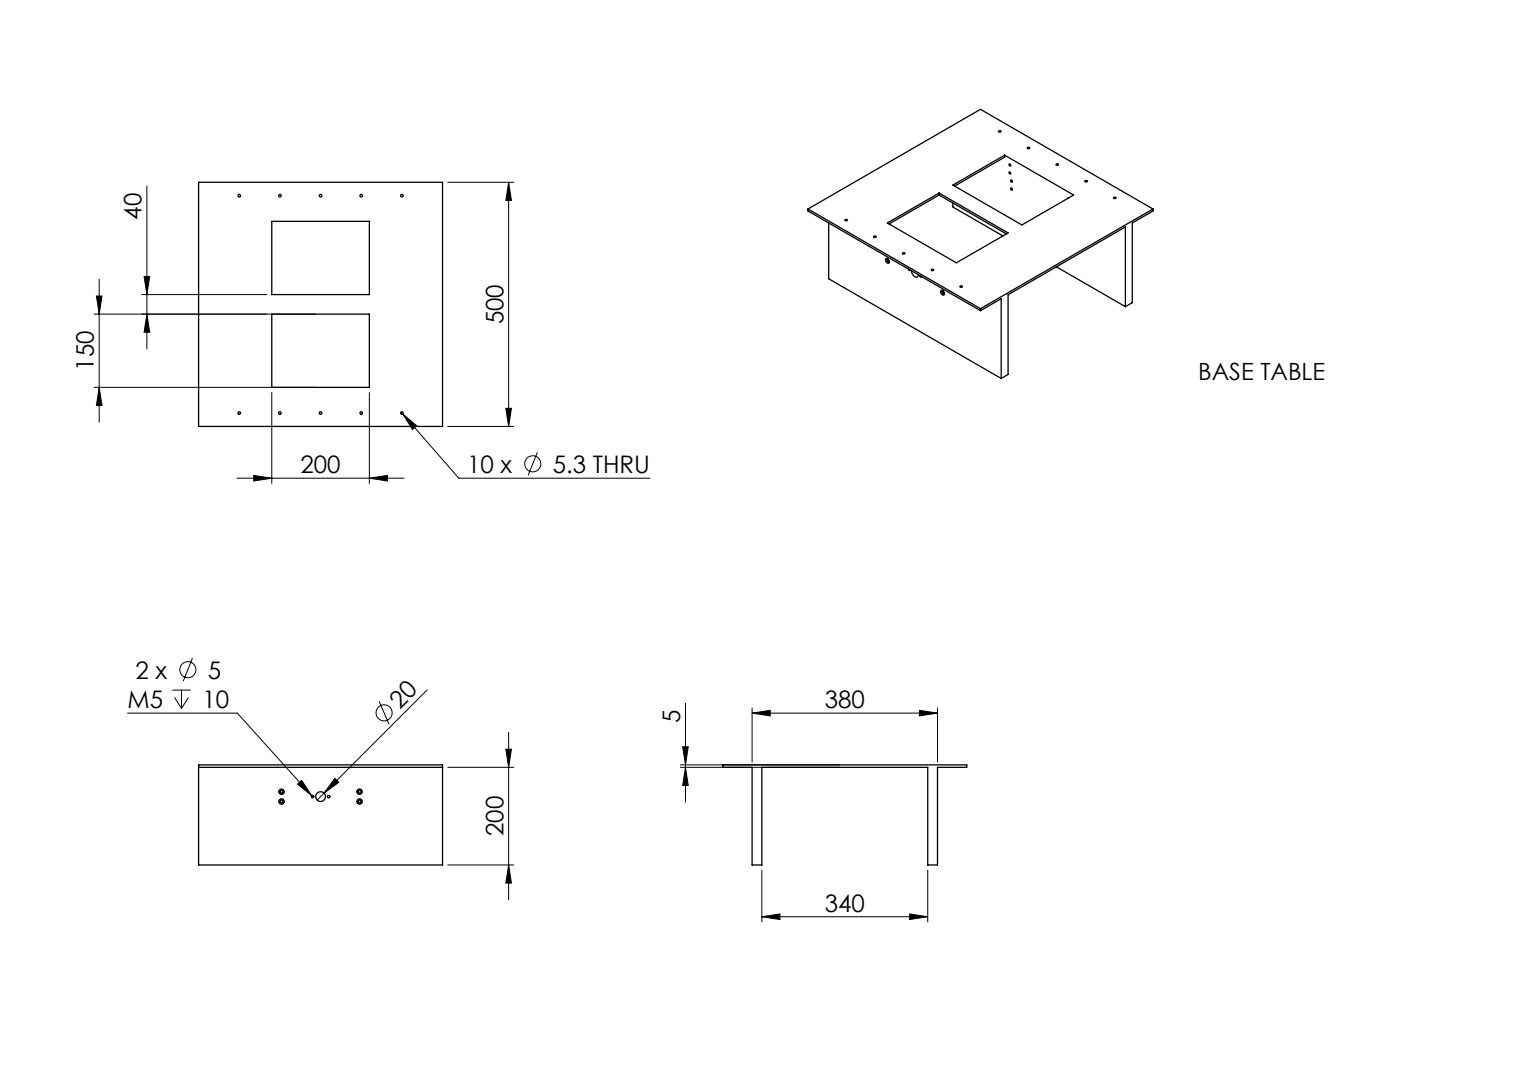
ISO-10303-21;
HEADER;
FILE_DESCRIPTION (('STEP AP214'),
    '1' );
FILE_NAME ('base table.step',
    '2026-10-24T13:33:06',
    ( '' ),
    ( '' ),
    'SwSTEP 2.0',
    'SolidWorks 2026',
    '' );
FILE_SCHEMA (( 'AUTOMOTIVE_DESIGN' ));
ENDSEC;

DATA;
#1=CARTESIAN_POINT ( 'NONE',  ( 53.33333333333330017, -25.00000000000000000, 222.5000000000000853 ) ) ;
#3=ORIENTED_EDGE ( 'NONE', *, *, #4024, .T. ) ;
#4=CARTESIAN_POINT ( 'NONE',  ( 302.6499999999999204, -75.00000000000008527, 169.9999999999999716 ) ) ;
#5=CARTESIAN_POINT ( 'NONE',  ( 136.6666666666666288, -20.00000000000000000, -219.8500000000001080 ) ) ;
#12=LINE ( 'NONE', #10262, #8342 ) ;
#13=LINE ( 'NONE', #14246, #12970 ) ;
#19=DIRECTION ( 'NONE',  ( 1.000000000000000000, 0.000000000000000000, 0.000000000000000000 ) ) ;
#22=CARTESIAN_POINT ( 'NONE',  ( 137.4999999999999432, -36.99999999999997868, -180.0000000000000000 ) ) ;
#29=CARTESIAN_POINT ( 'NONE',  ( 302.6499999999999204, -75.00000000000008527, 186.2999999999999829 ) ) ;
#36=ORIENTED_EDGE ( 'NONE', *, *, #2375, .F. ) ;
#40=ORIENTED_EDGE ( 'NONE', *, *, #13656, .T. ) ;
#44=DIRECTION ( 'NONE',  ( -0.000000000000000000, -0.000000000000000000, 1.000000000000000000 ) ) ;
#45=CARTESIAN_POINT ( 'NONE',  ( 386.6666666666666288, -20.00000000000000000, 225.1500000000000625 ) ) ;
#47=CARTESIAN_POINT ( 'NONE',  ( -30.00000000000002842, -25.00000000000000000, 250.0000000000000000 ) ) ;
#51=ORIENTED_EDGE ( 'NONE', *, *, #14217, .F. ) ;
#52=FACE_OUTER_BOUND ( 'NONE', #5422, .T. ) ;
#65=CARTESIAN_POINT ( 'NONE',  ( -30.00000000000002842, -20.00000000000000000, 250.0000000000000000 ) ) ;
#70=DIRECTION ( 'NONE',  ( 0.000000000000000000, 1.000000000000000000, 0.000000000000000000 ) ) ;
#76=LINE ( 'NONE', #7062, #6983 ) ;
#85=EDGE_CURVE ( 'NONE', #6756, #11518, #12060, .T. ) ;
#86=ADVANCED_FACE ( 'NONE', ( #14292 ), #14148, .F. ) ;
#90=ORIENTED_EDGE ( 'NONE', *, *, #8678, .T. ) ;
#96=ORIENTED_EDGE ( 'NONE', *, *, #5946, .F. ) ;
#107=LINE ( 'NONE', #12182, #1892 ) ;
#108=LINE ( 'NONE', #6679, #5937 ) ;
#111=CARTESIAN_POINT ( 'NONE',  ( 132.4999999999999432, -36.99999999999997868, -169.9999999999999716 ) ) ;
#113=CIRCLE ( 'NONE', #1517, 5.500000000000005329 ) ;
#119=CARTESIAN_POINT ( 'NONE',  ( 134.5000000000000000, -95.00000000000008527, 190.0000000000000000 ) ) ;
#122=LINE ( 'NONE', #2191, #4564 ) ;
#124=CARTESIAN_POINT ( 'NONE',  ( 142.6500000000000057, -95.00000000000008527, 190.0000000000000000 ) ) ;
#134=VECTOR ( 'NONE', #9384, 1000.000000000000000 ) ;
#138=VECTOR ( 'NONE', #5329, 1000.000000000000000 ) ;
#144=VECTOR ( 'NONE', #12485, 1000.000000000000000 ) ;
#164=EDGE_CURVE ( 'NONE', #13531, #14219, #11463, .T. ) ;
#173=PRODUCT ( 'base table', 'base table', '', ( #338 ) ) ;
#177=CIRCLE ( 'NONE', #2061, 2.500000000000002220 ) ;
#178=ORIENTED_EDGE ( 'NONE', *, *, #7566, .F. ) ;
#180=CARTESIAN_POINT ( 'NONE',  ( 299.9999999999999432, -95.00000000000008527, 190.0000000000000000 ) ) ;
#181=CARTESIAN_POINT ( 'NONE',  ( 302.6499999999999204, -95.00000000000008527, -186.2999999999999829 ) ) ;
#183=VECTOR ( 'NONE', #12816, 1000.000000000000000 ) ;
#186=DIRECTION ( 'NONE',  ( 1.000000000000000000, 0.000000000000000000, 0.000000000000000000 ) ) ;
#190=EDGE_LOOP ( 'NONE', ( #1618, #1963 ) ) ;
#192=CARTESIAN_POINT ( 'NONE',  ( 303.3333333333333144, -20.00000000000000000, -219.8500000000001080 ) ) ;
#193=ORIENTED_EDGE ( 'NONE', *, *, #7276, .F. ) ;
#195=CIRCLE ( 'NONE', #13619, 2.500000000000002220 ) ;
#196=EDGE_LOOP ( 'NONE', ( #178, #7479, #11699, #10408 ) ) ;
#197=DIRECTION ( 'NONE',  ( -0.000000000000000000, -0.000000000000000000, -1.000000000000000000 ) ) ;
#201=CARTESIAN_POINT ( 'NONE',  ( 294.4999999999999432, -75.00000000000008527, -190.0000000000000000 ) ) ;
#207=DIRECTION ( 'NONE',  ( 0.000000000000000000, -0.000000000000000000, 1.000000000000000000 ) ) ;
#211=ORIENTED_EDGE ( 'NONE', *, *, #1146, .F. ) ;
#223=LINE ( 'NONE', #12223, #5365 ) ;
#228=AXIS2_PLACEMENT_3D ( 'NONE', #3013, #14095, #2869 ) ;
#229=DIRECTION ( 'NONE',  ( -0.000000000000000000, -0.000000000000000000, -1.000000000000000000 ) ) ;
#234=EDGE_CURVE ( 'NONE', #10453, #9107, #4526, .T. ) ;
#244=ADVANCED_FACE ( 'NONE', ( #3220 ), #6544, .F. ) ;
#252=CARTESIAN_POINT ( 'NONE',  ( 307.5000000000000000, -56.99999999999997158, -180.0000000000000000 ) ) ;
#255=CARTESIAN_POINT ( 'NONE',  ( 119.9999999999999147, -20.00000000000000000, 19.99999999999998934 ) ) ;
#262=DIRECTION ( 'NONE',  ( -1.000000000000000000, 0.000000000000000000, 0.000000000000000000 ) ) ;
#265=ORIENTED_EDGE ( 'NONE', *, *, #11090, .F. ) ;
#266=EDGE_CURVE ( 'NONE', #11339, #3317, #13546, .T. ) ;
#267=CARTESIAN_POINT ( 'NONE',  ( 319.9999999999999432, -225.0010000000000048, 19.99999999999998934 ) ) ;
#268=ORIENTED_EDGE ( 'NONE', *, *, #5003, .F. ) ;
#279=ORIENTED_EDGE ( 'NONE', *, *, #5164, .T. ) ;
#288=DIRECTION ( 'NONE',  ( 0.000000000000000000, 0.000000000000000000, 1.000000000000000000 ) ) ;
#290=DIRECTION ( 'NONE',  ( -0.000000000000000000, 1.000000000000000000, -0.000000000000000000 ) ) ;
#293=EDGE_CURVE ( 'NONE', #12041, #2215, #4727, .T. ) ;
#295=CARTESIAN_POINT ( 'NONE',  ( 302.6499999999999204, -75.00000000000008527, 186.2999999999999829 ) ) ;
#299=DIRECTION ( 'NONE',  ( -0.000000000000000000, -0.000000000000000000, 1.000000000000000000 ) ) ;
#319=ORIENTED_EDGE ( 'NONE', *, *, #6736, .T. ) ;
#320=EDGE_LOOP ( 'NONE', ( #13311, #10317 ) ) ;
#322=AXIS2_PLACEMENT_3D ( 'NONE', #13350, #6899, #4588 ) ;
#325=CARTESIAN_POINT ( 'NONE',  ( 142.6500000000000057, -75.00000000000008527, 186.2999999999999829 ) ) ;
#326=EDGE_CURVE ( 'NONE', #2746, #3344, #2466, .T. ) ;
#328=VERTEX_POINT ( 'NONE', #3699 ) ;
#330=ORIENTED_EDGE ( 'NONE', *, *, #1288, .T. ) ;
#331=DIRECTION ( 'NONE',  ( 0.000000000000000000, 0.000000000000000000, 1.000000000000000000 ) ) ;
#336=CIRCLE ( 'NONE', #815, 5.500000000000005329 ) ;
#338=PRODUCT_CONTEXT ( 'NONE', #6572, 'mechanical' ) ;
#342=FACE_BOUND ( 'NONE', #10311, .T. ) ;
#347=ORIENTED_EDGE ( 'NONE', *, *, #12633, .T. ) ;
#357=DIRECTION ( 'NONE',  ( 1.000000000000000000, 0.000000000000000000, 0.000000000000000000 ) ) ;
#358=CARTESIAN_POINT ( 'NONE',  ( -30.00000000000002842, -225.0000000000000000, -169.9999999999999716 ) ) ;
#363=CIRCLE ( 'NONE', #6654, 2.649999999999985700 ) ;
#364=ORIENTED_EDGE ( 'NONE', *, *, #6973, .T. ) ;
#365=VECTOR ( 'NONE', #9606, 1000.000000000000000 ) ;
#366=VECTOR ( 'NONE', #12284, 1000.000000000000000 ) ;
#375=CARTESIAN_POINT ( 'NONE',  ( 132.4999999999999432, -56.99999999999997158, -180.0000000000000000 ) ) ;
#380=VECTOR ( 'NONE', #10926, 1000.000000000000000 ) ;
#381=DIRECTION ( 'NONE',  ( 0.000000000000000000, 0.000000000000000000, -1.000000000000000000 ) ) ;
#383=ADVANCED_FACE ( 'NONE', ( #52 ), #4580, .F. ) ;
#385=DIRECTION ( 'NONE',  ( -1.000000000000000000, 0.000000000000000000, 0.000000000000000000 ) ) ;
#390=CARTESIAN_POINT ( 'NONE',  ( 302.6499999999999204, -95.00000000000008527, -169.9999999999999716 ) ) ;
#391=CARTESIAN_POINT ( 'NONE',  ( 134.5000000000000000, -95.00000000000008527, -190.0000000000000000 ) ) ;
#398=EDGE_LOOP ( 'NONE', ( #3253, #13729, #3961, #12497 ) ) ;
#405=DIRECTION ( 'NONE',  ( 0.000000000000000000, 0.000000000000000000, -1.000000000000000000 ) ) ;
#409=FACE_BOUND ( 'NONE', #9655, .T. ) ;
#412=CARTESIAN_POINT ( 'NONE',  ( 140.0000000000000000, -75.00000000000008527, 186.2999999999999829 ) ) ;
#430=DIRECTION ( 'NONE',  ( -0.000000000000000000, -0.000000000000000000, 1.000000000000000000 ) ) ;
#434=EDGE_CURVE ( 'NONE', #8157, #4114, #1575, .T. ) ;
#439=( NAMED_UNIT ( * ) PLANE_ANGLE_UNIT ( ) SI_UNIT ( $, .RADIAN. ) );
#445=ORIENTED_EDGE ( 'NONE', *, *, #2431, .F. ) ;
#446=ADVANCED_FACE ( 'NONE', ( #13984, #8328 ), #12831, .F. ) ;
#453=AXIS2_PLACEMENT_3D ( 'NONE', #6130, #4839, #11360 ) ;
#464=CARTESIAN_POINT ( 'NONE',  ( 53.33333333333330017, -20.00000000000000000, -222.5000000000000853 ) ) ;
#474=ORIENTED_EDGE ( 'NONE', *, *, #10554, .T. ) ;
#481=CARTESIAN_POINT ( 'NONE',  ( 219.9999999999999716, -20.00000000000000000, -222.5000000000000853 ) ) ;
#504=EDGE_CURVE ( 'NONE', #1416, #12143, #787, .T. ) ;
#505=DIRECTION ( 'NONE',  ( 0.000000000000000000, 1.000000000000000000, 0.000000000000000000 ) ) ;
#511=DIRECTION ( 'NONE',  ( -1.000000000000000000, 0.000000000000000000, 0.000000000000000000 ) ) ;
#523=DIRECTION ( 'NONE',  ( 1.000000000000000000, 0.000000000000000000, 0.000000000000000000 ) ) ;
#525=DIRECTION ( 'NONE',  ( 1.000000000000000000, 0.000000000000000000, 0.000000000000000000 ) ) ;
#530=EDGE_CURVE ( 'NONE', #11552, #6716, #8218, .T. ) ;
#533=CYLINDRICAL_SURFACE ( 'NONE', #8092, 5.500000000000005329 ) ;
#541=CARTESIAN_POINT ( 'NONE',  ( 299.9999999999999432, -75.00000000000008527, -186.2999999999999829 ) ) ;
#552=AXIS2_PLACEMENT_3D ( 'NONE', #1164, #6764, #11129 ) ;
#563=SHAPE_DEFINITION_REPRESENTATION ( #6804, #2740 ) ;
#567=CIRCLE ( 'NONE', #11715, 5.500000000000005329 ) ;
#569=ORIENTED_EDGE ( 'NONE', *, *, #1110, .T. ) ;
#577=DIRECTION ( 'NONE',  ( -1.000000000000000000, 0.000000000000000000, 0.000000000000000000 ) ) ;
#580=CARTESIAN_POINT ( 'NONE',  ( 142.6500000000000057, -75.00000000000008527, 190.0000000000000000 ) ) ;
#581=CARTESIAN_POINT ( 'NONE',  ( -30.00000000000002842, -25.00000000000000000, -190.0000000000000000 ) ) ;
#582=VECTOR ( 'NONE', #10152, 1000.000000000000000 ) ;
#595=CIRCLE ( 'NONE', #10589, 2.649999999999985700 ) ;
#601=CIRCLE ( 'NONE', #4808, 5.500000000000005329 ) ;
#604=DIRECTION ( 'NONE',  ( 0.000000000000000000, 0.000000000000000000, -1.000000000000000000 ) ) ;
#614=EDGE_CURVE ( 'NONE', #1243, #10967, #14200, .T. ) ;
#624=FACE_OUTER_BOUND ( 'NONE', #10767, .T. ) ;
#626=CIRCLE ( 'NONE', #2277, 2.649999999999985700 ) ;
#627=EDGE_LOOP ( 'NONE', ( #3, #5676 ) ) ;
#630=FACE_OUTER_BOUND ( 'NONE', #8470, .T. ) ;
#634=VERTEX_POINT ( 'NONE', #11963 ) ;
#639=ADVANCED_FACE ( 'NONE', ( #12036 ), #6380, .T. ) ;
#641=CARTESIAN_POINT ( 'NONE',  ( 134.5000000000000000, -95.00000000000008527, 186.2999999999999829 ) ) ;
#647=EDGE_LOOP ( 'NONE', ( #6758, #1729, #6097, #8404 ) ) ;
#654=ORIENTED_EDGE ( 'NONE', *, *, #11946, .F. ) ;
#657=FACE_OUTER_BOUND ( 'NONE', #3143, .T. ) ;
#660=VECTOR ( 'NONE', #9403, 1000.000000000000000 ) ;
#665=EDGE_CURVE ( 'NONE', #10366, #9474, #11020, .T. ) ;
#668=CARTESIAN_POINT ( 'NONE',  ( 297.3499999999999659, -75.00000000000008527, 190.0000000000000000 ) ) ;
#670=CARTESIAN_POINT ( 'NONE',  ( 53.33333333333330017, -20.00000000000000000, 219.8500000000001080 ) ) ;
#677=ORIENTED_EDGE ( 'NONE', *, *, #85, .T. ) ;
#680=AXIS2_PLACEMENT_3D ( 'NONE', #9201, #13616, #5933 ) ;
#684=ADVANCED_FACE ( 'NONE', ( #12904 ), #1050, .F. ) ;
#687=CARTESIAN_POINT ( 'NONE',  ( 386.6666666666666288, -20.00000000000000000, -225.1500000000000625 ) ) ;
#691=DIRECTION ( 'NONE',  ( 1.000000000000000000, 0.000000000000000000, 0.000000000000000000 ) ) ;
#693=EDGE_CURVE ( 'NONE', #6913, #7861, #567, .T. ) ;
#699=ORIENTED_EDGE ( 'NONE', *, *, #13846, .F. ) ;
#701=VERTEX_POINT ( 'NONE', #8913 ) ;
#704=EDGE_CURVE ( 'NONE', #9413, #1808, #6868, .T. ) ;
#712=DIRECTION ( 'NONE',  ( -1.000000000000000000, 0.000000000000000000, 0.000000000000000000 ) ) ;
#715=ORIENTED_EDGE ( 'NONE', *, *, #13042, .T. ) ;
#716=EDGE_CURVE ( 'NONE', #12041, #2872, #7875, .T. ) ;
#721=CARTESIAN_POINT ( 'NONE',  ( 303.3333333333333144, -20.00000000000000000, 222.5000000000000853 ) ) ;
#724=ORIENTED_EDGE ( 'NONE', *, *, #9957, .F. ) ;
#732=DIRECTION ( 'NONE',  ( -1.000000000000000000, 0.000000000000000000, -0.000000000000000000 ) ) ;
#736=ORIENTED_EDGE ( 'NONE', *, *, #1947, .F. ) ;
#738=ORIENTED_EDGE ( 'NONE', *, *, #5484, .T. ) ;
#746=FACE_OUTER_BOUND ( 'NONE', #11832, .T. ) ;
#750=DIRECTION ( 'NONE',  ( -0.000000000000000000, 1.000000000000000000, -0.000000000000000000 ) ) ;
#751=ORIENTED_EDGE ( 'NONE', *, *, #4831, .F. ) ;
#761=LINE ( 'NONE', #8324, #11554 ) ;
#768=LINE ( 'NONE', #3270, #2096 ) ;
#770=VERTEX_POINT ( 'NONE', #6803 ) ;
#782=CARTESIAN_POINT ( 'NONE',  ( 307.5000000000000000, -56.99999999999997158, -169.9999999999999716 ) ) ;
#787=CIRCLE ( 'NONE', #4296, 2.649999999999985700 ) ;
#789=ORIENTED_EDGE ( 'NONE', *, *, #12859, .T. ) ;
#798=CARTESIAN_POINT ( 'NONE',  ( 319.9999999999999432, -20.00000000000000000, -169.9999999999999716 ) ) ;
#800=EDGE_CURVE ( 'NONE', #11046, #2569, #4631, .T. ) ;
#801=AXIS2_PLACEMENT_3D ( 'NONE', #6751, #6960, #5730 ) ;
#804=FACE_OUTER_BOUND ( 'NONE', #5648, .T. ) ;
#805=ORIENTED_EDGE ( 'NONE', *, *, #11640, .F. ) ;
#812=FACE_BOUND ( 'NONE', #4854, .T. ) ;
#815=AXIS2_PLACEMENT_3D ( 'NONE', #8559, #2026, #7322 ) ;
#816=DIRECTION ( 'NONE',  ( 0.000000000000000000, 1.000000000000000000, 0.000000000000000000 ) ) ;
#823=CARTESIAN_POINT ( 'NONE',  ( 134.9999999999999432, -56.99999999999997158, -181.5021515430661054 ) ) ;
#826=CARTESIAN_POINT ( 'NONE',  ( 302.6499999999999204, -95.00000000000008527, 186.2999999999999829 ) ) ;
#828=AXIS2_PLACEMENT_3D ( 'NONE', #1488, #13687, #385 ) ;
#832=CIRCLE ( 'NONE', #6862, 2.649999999999985700 ) ;
#833=FACE_OUTER_BOUND ( 'NONE', #7177, .T. ) ;
#835=CARTESIAN_POINT ( 'NONE',  ( 145.5000000000000284, -95.00000000000008527, -186.2999999999999829 ) ) ;
#840=VERTEX_POINT ( 'NONE', #10067 ) ;
#842=CARTESIAN_POINT ( 'NONE',  ( 470.0000000000000000, -25.00000000000000000, 190.0000000000000000 ) ) ;
#845=ORIENTED_EDGE ( 'NONE', *, *, #3733, .F. ) ;
#857=ORIENTED_EDGE ( 'NONE', *, *, #8071, .F. ) ;
#861=CARTESIAN_POINT ( 'NONE',  ( 142.6500000000000057, -75.00000000000008527, 169.9999999999999716 ) ) ;
#868=LINE ( 'NONE', #3158, #1741 ) ;
#871=EDGE_CURVE ( 'NONE', #1382, #840, #5112, .T. ) ;
#872=EDGE_CURVE ( 'NONE', #10300, #5386, #4179, .T. ) ;
#878=EDGE_CURVE ( 'NONE', #10453, #5579, #6146, .T. ) ;
#881=CYLINDRICAL_SURFACE ( 'NONE', #3412, 2.649999999999985700 ) ;
#887=CYLINDRICAL_SURFACE ( 'NONE', #1179, 5.500000000000005329 ) ;
#893=AXIS2_PLACEMENT_3D ( 'NONE', #8075, #11492, #13514 ) ;
#897=DIRECTION ( 'NONE',  ( -0.8571673013836870192, 1.049727191973306873E-16, 0.5150380737757234151 ) ) ;
#899=CYLINDRICAL_SURFACE ( 'NONE', #1302, 2.649999999999985700 ) ;
#908=FACE_OUTER_BOUND ( 'NONE', #5250, .T. ) ;
#912=ORIENTED_EDGE ( 'NONE', *, *, #1614, .T. ) ;
#918=PLANE ( 'NONE',  #2210 ) ;
#932=CARTESIAN_POINT ( 'NONE',  ( 206.0000000000000284, -85.00000000000007105, 190.0000000000000000 ) ) ;
#936=CIRCLE ( 'NONE', #6523, 2.649999999999985700 ) ;
#940=EDGE_CURVE ( 'NONE', #5316, #11325, #10663, .T. ) ;
#942=CARTESIAN_POINT ( 'NONE',  ( 303.3333333333333144, -20.00000000000000000, -222.5000000000000853 ) ) ;
#945=VECTOR ( 'NONE', #1140, 1000.000000000000000 ) ;
#947=EDGE_CURVE ( 'NONE', #11046, #13697, #12507, .T. ) ;
#948=DIRECTION ( 'NONE',  ( 0.000000000000000000, 0.000000000000000000, 1.000000000000000000 ) ) ;
#950=ADVANCED_FACE ( 'NONE', ( #2663 ), #533, .F. ) ;
#951=ORIENTED_EDGE ( 'NONE', *, *, #6482, .F. ) ;
#967=CARTESIAN_POINT ( 'NONE',  ( 386.6666666666666288, -25.00000000000000000, -225.1500000000000625 ) ) ;
#969=VECTOR ( 'NONE', #7214, 1000.000000000000000 ) ;
#982=CARTESIAN_POINT ( 'NONE',  ( 119.9999999999999147, -225.0010000000000048, 169.9999999999999716 ) ) ;
#989=DIRECTION ( 'NONE',  ( -0.000000000000000000, -0.000000000000000000, 1.000000000000000000 ) ) ;
#991=CARTESIAN_POINT ( 'NONE',  ( 305.0000000000000000, -56.99999999999997158, -180.0000000000000000 ) ) ;
#993=DIRECTION ( 'NONE',  ( -0.000000000000000000, 0.000000000000000000, 1.000000000000000000 ) ) ;
#995=CARTESIAN_POINT ( 'NONE',  ( 132.4999999999999432, -56.99999999999997158, -169.9999999999999716 ) ) ;
#1000=CARTESIAN_POINT ( 'NONE',  ( 307.5000000000000000, -36.99999999999997868, -180.0000000000000000 ) ) ;
#1001=EDGE_LOOP ( 'NONE', ( #951, #1693, #8534, #1264, #9691, #5453, #13384, #1955 ) ) ;
#1006=VERTEX_POINT ( 'NONE', #967 ) ;
#1009=DIRECTION ( 'NONE',  ( -0.000000000000000000, -0.000000000000000000, 1.000000000000000000 ) ) ;
#1012=CARTESIAN_POINT ( 'NONE',  ( 136.6666666666666288, -20.00000000000000000, 222.5000000000000853 ) ) ;
#1013=CARTESIAN_POINT ( 'NONE',  ( -30.00000000000002842, -25.00000000000000000, 169.9999999999999716 ) ) ;
#1020=VERTEX_POINT ( 'NONE', #9776 ) ;
#1023=EDGE_LOOP ( 'NONE', ( #4597, #2682 ) ) ;
#1025=PLANE ( 'NONE',  #13721 ) ;
#1027=AXIS2_PLACEMENT_3D ( 'NONE', #5838, #6852, #3593 ) ;
#1028=ORIENTED_EDGE ( 'NONE', *, *, #4301, .T. ) ;
#1035=AXIS2_PLACEMENT_3D ( 'NONE', #3051, #5502, #14059 ) ;
#1048=ORIENTED_EDGE ( 'NONE', *, *, #6214, .T. ) ;
#1050=CYLINDRICAL_SURFACE ( 'NONE', #1035, 2.649999999999985700 ) ;
#1053=DIRECTION ( 'NONE',  ( -0.000000000000000000, 0.000000000000000000, -1.000000000000000000 ) ) ;
#1056=EDGE_CURVE ( 'NONE', #13697, #10145, #8756, .T. ) ;
#1065=DIRECTION ( 'NONE',  ( -0.000000000000000000, -1.000000000000000000, -0.000000000000000000 ) ) ;
#1066=AXIS2_PLACEMENT_3D ( 'NONE', #12203, #2342, #2270 ) ;
#1068=CYLINDRICAL_SURFACE ( 'NONE', #8248, 5.500000000000005329 ) ;
#1072=ORIENTED_EDGE ( 'NONE', *, *, #85, .F. ) ;
#1075=AXIS2_PLACEMENT_3D ( 'NONE', #7410, #2850, #7263 ) ;
#1080=EDGE_CURVE ( 'NONE', #14253, #2215, #14042, .T. ) ;
#1086=CIRCLE ( 'NONE', #12451, 2.500000000000002220 ) ;
#1091=( LENGTH_UNIT ( ) NAMED_UNIT ( * ) SI_UNIT ( .MILLI., .METRE. ) );
#1095=DIRECTION ( 'NONE',  ( 0.000000000000000000, 0.000000000000000000, -1.000000000000000000 ) ) ;
#1096=ORIENTED_EDGE ( 'NONE', *, *, #3247, .F. ) ;
#1101=CYLINDRICAL_SURFACE ( 'NONE', #5026, 2.649999999999985700 ) ;
#1109=DIRECTION ( 'NONE',  ( -0.000000000000000000, 1.000000000000000000, -0.000000000000000000 ) ) ;
#1110=EDGE_CURVE ( 'NONE', #8867, #8759, #4189, .T. ) ;
#1117=ORIENTED_EDGE ( 'NONE', *, *, #9700, .F. ) ;
#1118=LINE ( 'NONE', #2643, #11978 ) ;
#1120=DIRECTION ( 'NONE',  ( -0.000000000000000000, -0.000000000000000000, -1.000000000000000000 ) ) ;
#1125=VERTEX_POINT ( 'NONE', #823 ) ;
#1131=ORIENTED_EDGE ( 'NONE', *, *, #12517, .F. ) ;
#1132=ORIENTED_EDGE ( 'NONE', *, *, #2253, .T. ) ;
#1134=DIRECTION ( 'NONE',  ( -1.000000000000000000, 0.000000000000000000, 0.000000000000000000 ) ) ;
#1138=AXIS2_PLACEMENT_3D ( 'NONE', #13702, #10598, #12689 ) ;
#1140=DIRECTION ( 'NONE',  ( -0.000000000000000000, 1.000000000000000000, -0.000000000000000000 ) ) ;
#1141=DIRECTION ( 'NONE',  ( -0.000000000000000000, -0.000000000000000000, 1.000000000000000000 ) ) ;
#1146=EDGE_CURVE ( 'NONE', #10315, #11952, #6039, .T. ) ;
#1152=VECTOR ( 'NONE', #8133, 1000.000000000000000 ) ;
#1154=EDGE_CURVE ( 'NONE', #3317, #2814, #8816, .T. ) ;
#1159=VECTOR ( 'NONE', #2534, 1000.000000000000000 ) ;
#1164=CARTESIAN_POINT ( 'NONE',  ( 140.0000000000000000, -75.00000000000008527, 186.2999999999999829 ) ) ;
#1168=ADVANCED_FACE ( 'NONE', ( #13249 ), #9988, .F. ) ;
#1169=EDGE_CURVE ( 'NONE', #1125, #9107, #13723, .T. ) ;
#1172=EDGE_LOOP ( 'NONE', ( #1315, #8576 ) ) ;
#1173=ADVANCED_FACE ( 'NONE', ( #9235, #6910 ), #3583, .F. ) ;
#1176=ORIENTED_EDGE ( 'NONE', *, *, #293, .F. ) ;
#1179=AXIS2_PLACEMENT_3D ( 'NONE', #10929, #10718, #7581 ) ;
#1181=DIRECTION ( 'NONE',  ( -0.000000000000000000, 0.000000000000000000, 1.000000000000000000 ) ) ;
#1183=CARTESIAN_POINT ( 'NONE',  ( 294.4999999999999432, -75.00000000000008527, -190.0000000000000000 ) ) ;
#1186=DIRECTION ( 'NONE',  ( -0.000000000000000000, 1.000000000000000000, -0.000000000000000000 ) ) ;
#1187=CARTESIAN_POINT ( 'NONE',  ( 299.9999999999999432, -75.00000000000008527, -186.2999999999999829 ) ) ;
#1189=LINE ( 'NONE', #5768, #6517 ) ;
#1192=CARTESIAN_POINT ( 'NONE',  ( 470.0000000000000000, -25.00000000000000000, 250.0000000000000000 ) ) ;
#1193=ADVANCED_FACE ( 'NONE', ( #9918 ), #9336, .F. ) ;
#1194=ORIENTED_EDGE ( 'NONE', *, *, #2773, .T. ) ;
#1195=CARTESIAN_POINT ( 'NONE',  ( 305.4999999999999432, -95.00000000000008527, 186.2999999999999829 ) ) ;
#1199=FACE_OUTER_BOUND ( 'NONE', #9157, .T. ) ;
#1202=AXIS2_PLACEMENT_3D ( 'NONE', #11836, #12995, #2993 ) ;
#1203=ORIENTED_EDGE ( 'NONE', *, *, #5421, .T. ) ;
#1205=( NAMED_UNIT ( * ) SI_UNIT ( $, .STERADIAN. ) SOLID_ANGLE_UNIT ( ) );
#1210=ORIENTED_EDGE ( 'NONE', *, *, #9443, .F. ) ;
#1215=DIRECTION ( 'NONE',  ( -0.000000000000000000, -0.000000000000000000, 1.000000000000000000 ) ) ;
#1216=DIRECTION ( 'NONE',  ( -0.000000000000000000, -0.000000000000000000, 1.000000000000000000 ) ) ;
#1220=DIRECTION ( 'NONE',  ( 0.000000000000000000, 0.000000000000000000, -1.000000000000000000 ) ) ;
#1224=ORIENTED_EDGE ( 'NONE', *, *, #3247, .T. ) ;
#1226=ORIENTED_EDGE ( 'NONE', *, *, #3673, .F. ) ;
#1230=ORIENTED_EDGE ( 'NONE', *, *, #4069, .T. ) ;
#1231=PLANE ( 'NONE',  #3603 ) ;
#1243=VERTEX_POINT ( 'NONE', #9159 ) ;
#1252=EDGE_CURVE ( 'NONE', #3125, #6716, #11626, .T. ) ;
#1260=CARTESIAN_POINT ( 'NONE',  ( 136.6666666666666288, -25.00000000000000000, 222.5000000000000853 ) ) ;
#1264=ORIENTED_EDGE ( 'NONE', *, *, #4414, .T. ) ;
#1266=DIRECTION ( 'NONE',  ( -1.000000000000000000, 0.000000000000000000, 0.000000000000000000 ) ) ;
#1281=LINE ( 'NONE', #5721, #945 ) ;
#1286=AXIS2_PLACEMENT_3D ( 'NONE', #9219, #6100, #8120 ) ;
#1287=ORIENTED_EDGE ( 'NONE', *, *, #13354, .T. ) ;
#1288=EDGE_CURVE ( 'NONE', #1020, #2372, #9042, .T. ) ;
#1291=CARTESIAN_POINT ( 'NONE',  ( 470.0000000000000000, -20.00000000000000000, 250.0000000000000000 ) ) ;
#1293=ORIENTED_EDGE ( 'NONE', *, *, #9936, .T. ) ;
#1295=VECTOR ( 'NONE', #505, 1000.000000000000000 ) ;
#1297=DIRECTION ( 'NONE',  ( 0.000000000000000000, 0.000000000000000000, -1.000000000000000000 ) ) ;
#1302=AXIS2_PLACEMENT_3D ( 'NONE', #4049, #7521, #1864 ) ;
#1306=CARTESIAN_POINT ( 'NONE',  ( -30.00000000000002842, -25.00000000000000000, 250.0000000000000000 ) ) ;
#1313=ORIENTED_EDGE ( 'NONE', *, *, #13261, .T. ) ;
#1315=ORIENTED_EDGE ( 'NONE', *, *, #12071, .F. ) ;
#1323=EDGE_CURVE ( 'NONE', #3167, #3720, #9507, .T. ) ;
#1333=DIRECTION ( 'NONE',  ( 0.000000000000000000, 1.000000000000000000, 0.000000000000000000 ) ) ;
#1343=EDGE_CURVE ( 'NONE', #6665, #8094, #10619, .T. ) ;
#1348=EDGE_LOOP ( 'NONE', ( #3565, #1722 ) ) ;
#1349=CARTESIAN_POINT ( 'NONE',  ( 203.5000000000000000, -85.00000000000007105, 180.0000000000000000 ) ) ;
#1352=ORIENTED_EDGE ( 'NONE', *, *, #13379, .F. ) ;
#1369=ORIENTED_EDGE ( 'NONE', *, *, #12633, .F. ) ;
#1370=FACE_OUTER_BOUND ( 'NONE', #7900, .T. ) ;
#1371=ORIENTED_EDGE ( 'NONE', *, *, #13161, .F. ) ;
#1372=CIRCLE ( 'NONE', #11351, 2.649999999999985700 ) ;
#1373=DIRECTION ( 'NONE',  ( -0.000000000000000000, -0.000000000000000000, 1.000000000000000000 ) ) ;
#1374=CARTESIAN_POINT ( 'NONE',  ( 299.9999999999999432, -95.00000000000008527, 186.2999999999999829 ) ) ;
#1380=CARTESIAN_POINT ( 'NONE',  ( 238.9999999999999432, -85.00000000000007105, 190.0000000000000000 ) ) ;
#1381=VERTEX_POINT ( 'NONE', #6113 ) ;
#1382=VERTEX_POINT ( 'NONE', #5186 ) ;
#1389=ORIENTED_EDGE ( 'NONE', *, *, #13899, .T. ) ;
#1390=DIRECTION ( 'NONE',  ( 1.000000000000000000, 0.000000000000000000, 0.000000000000000000 ) ) ;
#1397=FACE_OUTER_BOUND ( 'NONE', #9178, .T. ) ;
#1404=DIRECTION ( 'NONE',  ( -1.000000000000000000, 0.000000000000000000, 0.000000000000000000 ) ) ;
#1407=EDGE_LOOP ( 'NONE', ( #8578, #7757, #9815, #9066 ) ) ;
#1408=AXIS2_PLACEMENT_3D ( 'NONE', #6574, #5477, #9911 ) ;
#1415=EDGE_CURVE ( 'NONE', #6044, #3377, #11120, .T. ) ;
#1416=VERTEX_POINT ( 'NONE', #3365 ) ;
#1418=AXIS2_PLACEMENT_3D ( 'NONE', #10970, #3355, #2105 ) ;
#1422=EDGE_LOOP ( 'NONE', ( #10256, #6078 ) ) ;
#1442=CARTESIAN_POINT ( 'NONE',  ( 470.0000000000000000, -25.00000000000000000, 250.0000000000000000 ) ) ;
#1447=DIRECTION ( 'NONE',  ( -1.000000000000000000, 0.000000000000000000, 0.000000000000000000 ) ) ;
#1448=VERTEX_POINT ( 'NONE', #12062 ) ;
#1449=CYLINDRICAL_SURFACE ( 'NONE', #13340, 2.649999999999985700 ) ;
#1451=DIRECTION ( 'NONE',  ( 0.000000000000000000, 0.000000000000000000, -1.000000000000000000 ) ) ;
#1452=VERTEX_POINT ( 'NONE', #861 ) ;
#1454=DIRECTION ( 'NONE',  ( 0.000000000000000000, 0.000000000000000000, 1.000000000000000000 ) ) ;
#1456=FACE_BOUND ( 'NONE', #10648, .T. ) ;
#1460=ADVANCED_FACE ( 'NONE', ( #5530 ), #8865, .F. ) ;
#1466=DIRECTION ( 'NONE',  ( -0.000000000000000000, -0.000000000000000000, 1.000000000000000000 ) ) ;
#1473=CARTESIAN_POINT ( 'NONE',  ( 53.33333333333330017, -20.00000000000000000, -225.1500000000000625 ) ) ;
#1478=ADVANCED_FACE ( 'NONE', ( #2117 ), #2261, .F. ) ;
#1479=LINE ( 'NONE', #10272, #3517 ) ;
#1487=EDGE_LOOP ( 'NONE', ( #13050, #13231, #569, #1131 ) ) ;
#1488=CARTESIAN_POINT ( 'NONE',  ( 140.0000000000000000, -95.00000000000008527, -190.0000000000000000 ) ) ;
#1493=LINE ( 'NONE', #2671, #6042 ) ;
#1499=ORIENTED_EDGE ( 'NONE', *, *, #14078, .F. ) ;
#1501=EDGE_CURVE ( 'NONE', #7291, #7986, #5623, .T. ) ;
#1508=ORIENTED_EDGE ( 'NONE', *, *, #7566, .T. ) ;
#1509=DIRECTION ( 'NONE',  ( 0.000000000000000000, 0.000000000000000000, -1.000000000000000000 ) ) ;
#1510=ORIENTED_EDGE ( 'NONE', *, *, #1288, .F. ) ;
#1513=DIRECTION ( 'NONE',  ( -1.000000000000000000, 0.000000000000000000, 0.000000000000000000 ) ) ;
#1517=AXIS2_PLACEMENT_3D ( 'NONE', #11311, #5715, #11102 ) ;
#1522=DIRECTION ( 'NONE',  ( -1.000000000000000000, 0.000000000000000000, 0.000000000000000000 ) ) ;
#1531=EDGE_LOOP ( 'NONE', ( #3203, #13066, #4904 ) ) ;
#1539=DIRECTION ( 'NONE',  ( 0.000000000000000000, 1.000000000000000000, 0.000000000000000000 ) ) ;
#1541=DIRECTION ( 'NONE',  ( 0.000000000000000000, 0.000000000000000000, 1.000000000000000000 ) ) ;
#1550=ORIENTED_EDGE ( 'NONE', *, *, #2851, .F. ) ;
#1557=AXIS2_PLACEMENT_3D ( 'NONE', #464, #13905, #5078 ) ;
#1558=VERTEX_POINT ( 'NONE', #119 ) ;
#1563=FACE_BOUND ( 'NONE', #12336, .T. ) ;
#1568=LINE ( 'NONE', #1643, #3080 ) ;
#1573=EDGE_LOOP ( 'NONE', ( #1925, #12567, #6022, #193 ) ) ;
#1575=LINE ( 'NONE', #2902, #5911 ) ;
#1578=DIRECTION ( 'NONE',  ( 0.000000000000000000, 0.000000000000000000, 1.000000000000000000 ) ) ;
#1584=FACE_OUTER_BOUND ( 'NONE', #8667, .T. ) ;
#1595=ORIENTED_EDGE ( 'NONE', *, *, #3891, .F. ) ;
#1596=AXIS2_PLACEMENT_3D ( 'NONE', #12454, #5918, #11436 ) ;
#1597=EDGE_CURVE ( 'NONE', #3594, #13983, #12100, .T. ) ;
#1602=EDGE_CURVE ( 'NONE', #1381, #10838, #1911, .T. ) ;
#1603=EDGE_LOOP ( 'NONE', ( #9481, #9467, #7447, #1731 ) ) ;
#1605=ORIENTED_EDGE ( 'NONE', *, *, #12867, .T. ) ;
#1608=CARTESIAN_POINT ( 'NONE',  ( 0.000000000000000000, 0.000000000000000000, 250.0000000000000000 ) ) ;
#1610=EDGE_CURVE ( 'NONE', #328, #11751, #2402, .T. ) ;
#1614=EDGE_CURVE ( 'NONE', #12208, #6338, #5662, .T. ) ;
#1618=ORIENTED_EDGE ( 'NONE', *, *, #5421, .F. ) ;
#1622=DIRECTION ( 'NONE',  ( -0.000000000000000000, -0.000000000000000000, -1.000000000000000000 ) ) ;
#1629=AXIS2_PLACEMENT_3D ( 'NONE', #8903, #3394, #3334 ) ;
#1638=CIRCLE ( 'NONE', #1408, 2.649999999999985700 ) ;
#1643=CARTESIAN_POINT ( 'NONE',  ( 386.6666666666666288, -20.00000000000000000, -225.1500000000000625 ) ) ;
#1658=ORIENTED_EDGE ( 'NONE', *, *, #3196, .F. ) ;
#1662=VERTEX_POINT ( 'NONE', #325 ) ;
#1665=CARTESIAN_POINT ( 'NONE',  ( 469.9999999999998863, -25.00000000000000000, 169.9999999999999716 ) ) ;
#1668=VECTOR ( 'NONE', #2684, 1000.000000000000000 ) ;
#1672=EDGE_LOOP ( 'NONE', ( #11529, #10002, #6110, #12494 ) ) ;
#1676=CIRCLE ( 'NONE', #9804, 5.500000000000005329 ) ;
#1677=VERTEX_POINT ( 'NONE', #10297 ) ;
#1678=CARTESIAN_POINT ( 'NONE',  ( 206.0000000000000284, -85.00000000000007105, 180.0000000000000000 ) ) ;
#1680=ORIENTED_EDGE ( 'NONE', *, *, #11034, .F. ) ;
#1686=PLANE ( 'NONE',  #10340 ) ;
#1687=EDGE_CURVE ( 'NONE', #8236, #6756, #13958, .T. ) ;
#1689=DIRECTION ( 'NONE',  ( -1.000000000000000000, 0.000000000000000000, 0.000000000000000000 ) ) ;
#1693=ORIENTED_EDGE ( 'NONE', *, *, #13590, .F. ) ;
#1696=LINE ( 'NONE', #8592, #14186 ) ;
#1707=CARTESIAN_POINT ( 'NONE',  ( 219.9999999999999716, -20.00000000000000000, -219.8500000000001080 ) ) ;
#1711=ADVANCED_FACE ( 'NONE', ( #9069 ), #13491, .F. ) ;
#1713=ORIENTED_EDGE ( 'NONE', *, *, #6768, .T. ) ;
#1714=FACE_BOUND ( 'NONE', #7568, .T. ) ;
#1717=CARTESIAN_POINT ( 'NONE',  ( 302.6499999999999204, -75.00000000000008527, -190.0000000000000000 ) ) ;
#1721=CARTESIAN_POINT ( 'NONE',  ( 302.6499999999999204, -95.00000000000008527, 169.9999999999999716 ) ) ;
#1722=ORIENTED_EDGE ( 'NONE', *, *, #5484, .F. ) ;
#1724=ORIENTED_EDGE ( 'NONE', *, *, #11002, .T. ) ;
#1727=AXIS2_PLACEMENT_3D ( 'NONE', #10900, #5387, #9814 ) ;
#1728=CIRCLE ( 'NONE', #7063, 5.500000000000005329 ) ;
#1729=ORIENTED_EDGE ( 'NONE', *, *, #11443, .F. ) ;
#1731=ORIENTED_EDGE ( 'NONE', *, *, #13950, .F. ) ;
#1733=DIRECTION ( 'NONE',  ( -0.000000000000000000, -0.000000000000000000, -1.000000000000000000 ) ) ;
#1734=ORIENTED_EDGE ( 'NONE', *, *, #8640, .F. ) ;
#1740=FACE_BOUND ( 'NONE', #8515, .T. ) ;
#1741=VECTOR ( 'NONE', #6342, 1000.000000000000000 ) ;
#1742=ORIENTED_EDGE ( 'NONE', *, *, #293, .T. ) ;
#1749=ORIENTED_EDGE ( 'NONE', *, *, #9790, .T. ) ;
#1753=FACE_BOUND ( 'NONE', #3200, .T. ) ;
#1754=AXIS2_PLACEMENT_3D ( 'NONE', #8777, #4361, #2243 ) ;
#1756=CARTESIAN_POINT ( 'NONE',  ( 140.0000000000000000, -75.00000000000008527, -186.2999999999999829 ) ) ;
#1759=ORIENTED_EDGE ( 'NONE', *, *, #11011, .F. ) ;
#1767=CYLINDRICAL_SURFACE ( 'NONE', #6316, 2.500000000000002220 ) ;
#1768=DIRECTION ( 'NONE',  ( 1.000000000000000000, 0.000000000000000000, 0.000000000000000000 ) ) ;
#1769=AXIS2_PLACEMENT_3D ( 'NONE', #10108, #5900, #4680 ) ;
#1776=CARTESIAN_POINT ( 'NONE',  ( 386.6666666666666288, -20.00000000000000000, -222.5000000000000853 ) ) ;
#1780=AXIS2_PLACEMENT_3D ( 'NONE', #6415, #6701, #9827 ) ;
#1785=CARTESIAN_POINT ( 'NONE',  ( 119.9999999999999147, -20.00000000000000000, -19.99999999999998934 ) ) ;
#1795=CARTESIAN_POINT ( 'NONE',  ( 303.3333333333333144, -25.00000000000000000, 222.5000000000000853 ) ) ;
#1801=CIRCLE ( 'NONE', #13382, 2.649999999999985700 ) ;
#1803=EDGE_CURVE ( 'NONE', #11373, #11952, #13987, .T. ) ;
#1808=VERTEX_POINT ( 'NONE', #13773 ) ;
#1815=CIRCLE ( 'NONE', #893, 2.500000000000002220 ) ;
#1820=DIRECTION ( 'NONE',  ( 1.000000000000000000, 0.000000000000000000, 0.000000000000000000 ) ) ;
#1826=DIRECTION ( 'NONE',  ( 0.8571673013836870192, 0.000000000000000000, 0.5150380737757234151 ) ) ;
#1827=EDGE_CURVE ( 'NONE', #2165, #7848, #10425, .T. ) ;
#1828=ORIENTED_EDGE ( 'NONE', *, *, #9026, .F. ) ;
#1832=DIRECTION ( 'NONE',  ( -1.000000000000000000, 0.000000000000000000, 0.000000000000000000 ) ) ;
#1839=VERTEX_POINT ( 'NONE', #7173 ) ;
#1847=FACE_OUTER_BOUND ( 'NONE', #5801, .T. ) ;
#1849=AXIS2_PLACEMENT_3D ( 'NONE', #7156, #3900, #4772 ) ;
#1851=VECTOR ( 'NONE', #10499, 1000.000000000000000 ) ;
#1855=FACE_OUTER_BOUND ( 'NONE', #9978, .T. ) ;
#1862=FACE_BOUND ( 'NONE', #627, .T. ) ;
#1864=DIRECTION ( 'NONE',  ( 0.000000000000000000, 0.000000000000000000, 1.000000000000000000 ) ) ;
#1866=VECTOR ( 'NONE', #11220, 1000.000000000000000 ) ;
#1868=EDGE_CURVE ( 'NONE', #5579, #9676, #6023, .T. ) ;
#1874=AXIS2_PLACEMENT_3D ( 'NONE', #7138, #430, #13658 ) ;
#1876=CARTESIAN_POINT ( 'NONE',  ( 305.4999999999999432, -75.00000000000008527, 186.2999999999999829 ) ) ;
#1882=EDGE_CURVE ( 'NONE', #10615, #4007, #6455, .T. ) ;
#1886=DIRECTION ( 'NONE',  ( -0.000000000000000000, -0.000000000000000000, 1.000000000000000000 ) ) ;
#1888=EDGE_LOOP ( 'NONE', ( #4304, #13023 ) ) ;
#1892=VECTOR ( 'NONE', #2249, 1000.000000000000000 ) ;
#1906=ORIENTED_EDGE ( 'NONE', *, *, #6410, .T. ) ;
#1910=LINE ( 'NONE', #1013, #138 ) ;
#1911=CIRCLE ( 'NONE', #9558, 2.649999999999985700 ) ;
#1920=CARTESIAN_POINT ( 'NONE',  ( -30.00000000000002842, -225.0000000000000000, 190.0000000000000000 ) ) ;
#1925=ORIENTED_EDGE ( 'NONE', *, *, #12785, .F. ) ;
#1926=CARTESIAN_POINT ( 'NONE',  ( 299.9999999999999432, -75.00000000000008527, 190.0000000000000000 ) ) ;
#1927=LINE ( 'NONE', #5283, #4858 ) ;
#1931=EDGE_LOOP ( 'NONE', ( #1371, #6287 ) ) ;
#1933=DIRECTION ( 'NONE',  ( 1.000000000000000000, 0.000000000000000000, 0.000000000000000000 ) ) ;
#1934=DIRECTION ( 'NONE',  ( 0.000000000000000000, 0.000000000000000000, -1.000000000000000000 ) ) ;
#1935=ADVANCED_FACE ( 'NONE', ( #908 ), #6526, .F. ) ;
#1944=ORIENTED_EDGE ( 'NONE', *, *, #5173, .F. ) ;
#1945=CARTESIAN_POINT ( 'NONE',  ( -30.00000000000002842, -225.0000000000000000, -190.0000000000000000 ) ) ;
#1947=EDGE_CURVE ( 'NONE', #6913, #4174, #10811, .T. ) ;
#1951=ORIENTED_EDGE ( 'NONE', *, *, #14113, .T. ) ;
#1955=ORIENTED_EDGE ( 'NONE', *, *, #9788, .F. ) ;
#1963=ORIENTED_EDGE ( 'NONE', *, *, #5243, .F. ) ;
#1966=VECTOR ( 'NONE', #6891, 1000.000000000000000 ) ;
#1983=ADVANCED_FACE ( 'NONE', ( #2021 ), #7673, .T. ) ;
#1986=ADVANCED_FACE ( 'NONE', ( #9934 ), #5229, .F. ) ;
#1989=ORIENTED_EDGE ( 'NONE', *, *, #10530, .F. ) ;
#1992=ORIENTED_EDGE ( 'NONE', *, *, #5529, .T. ) ;
#1995=CARTESIAN_POINT ( 'NONE',  ( -30.00000000000002842, -25.00000000000000000, 169.9999999999999716 ) ) ;
#1997=DIRECTION ( 'NONE',  ( -1.000000000000000000, 0.000000000000000000, 0.000000000000000000 ) ) ;
#1999=ORIENTED_EDGE ( 'NONE', *, *, #7259, .T. ) ;
#2002=LINE ( 'NONE', #6441, #9050 ) ;
#2016=CIRCLE ( 'NONE', #4589, 2.649999999999985700 ) ;
#2018=CIRCLE ( 'NONE', #3199, 5.500000000000005329 ) ;
#2020=DIRECTION ( 'NONE',  ( 0.8571673013836870192, 0.000000000000000000, 0.5150380737757234151 ) ) ;
#2021=FACE_OUTER_BOUND ( 'NONE', #12943, .T. ) ;
#2022=EDGE_CURVE ( 'NONE', #11916, #14253, #9557, .T. ) ;
#2023=CIRCLE ( 'NONE', #1075, 2.649999999999985700 ) ;
#2024=EDGE_LOOP ( 'NONE', ( #7453, #13722, #2432, #3268 ) ) ;
#2026=DIRECTION ( 'NONE',  ( -0.000000000000000000, -0.000000000000000000, -1.000000000000000000 ) ) ;
#2028=CARTESIAN_POINT ( 'NONE',  ( 307.5000000000000000, -36.99999999999997868, -169.9999999999999716 ) ) ;
#2035=EDGE_CURVE ( 'NONE', #10043, #13274, #4113, .T. ) ;
#2036=VERTEX_POINT ( 'NONE', #3816 ) ;
#2037=ORIENTED_EDGE ( 'NONE', *, *, #1146, .T. ) ;
#2039=ORIENTED_EDGE ( 'NONE', *, *, #8435, .T. ) ;
#2042=ORIENTED_EDGE ( 'NONE', *, *, #13545, .F. ) ;
#2053=CIRCLE ( 'NONE', #6478, 5.500000000000005329 ) ;
#2055=EDGE_CURVE ( 'NONE', #11403, #13651, #6360, .T. ) ;
#2057=EDGE_LOOP ( 'NONE', ( #2612, #13253 ) ) ;
#2061=AXIS2_PLACEMENT_3D ( 'NONE', #5443, #1215, #5612 ) ;
#2067=CARTESIAN_POINT ( 'NONE',  ( 119.9999999999999147, -20.00000000000000000, -169.9999999999999716 ) ) ;
#2082=EDGE_LOOP ( 'NONE', ( #4217, #8427 ) ) ;
#2087=AXIS2_PLACEMENT_3D ( 'NONE', #5034, #8498, #4079 ) ;
#2092=DIRECTION ( 'NONE',  ( -1.000000000000000000, 0.000000000000000000, 0.000000000000000000 ) ) ;
#2096=VECTOR ( 'NONE', #7672, 1000.000000000000000 ) ;
#2105=DIRECTION ( 'NONE',  ( 0.000000000000000000, 0.000000000000000000, 1.000000000000000000 ) ) ;
#2106=CARTESIAN_POINT ( 'NONE',  ( 469.9999999999998863, -225.0000000000000000, 190.0000000000000000 ) ) ;
#2109=CARTESIAN_POINT ( 'NONE',  ( 140.0000000000000000, -75.00000000000008527, -169.9999999999999716 ) ) ;
#2111=EDGE_LOOP ( 'NONE', ( #2285, #9909, #3142, #4212 ) ) ;
#2117=FACE_OUTER_BOUND ( 'NONE', #11878, .T. ) ;
#2120=LINE ( 'NONE', #932, #12211 ) ;
#2121=VERTEX_POINT ( 'NONE', #6281 ) ;
#2122=EDGE_CURVE ( 'NONE', #13543, #2746, #10722, .T. ) ;
#2130=DIRECTION ( 'NONE',  ( -0.000000000000000000, -1.000000000000000000, -0.000000000000000000 ) ) ;
#2134=AXIS2_PLACEMENT_3D ( 'NONE', #4026, #2935, #1689 ) ;
#2139=VECTOR ( 'NONE', #1826, 1000.000000000000000 ) ;
#2142=PRODUCT_DEFINITION ( 'UNKNOWN', '', #4249, #14046 ) ;
#2144=EDGE_LOOP ( 'NONE', ( #11697, #1713, #2037, #6971 ) ) ;
#2157=DIRECTION ( 'NONE',  ( 1.000000000000000000, 0.000000000000000000, 0.000000000000000000 ) ) ;
#2159=LINE ( 'NONE', #4968, #8486 ) ;
#2161=DIRECTION ( 'NONE',  ( -1.000000000000000000, 0.000000000000000000, -0.000000000000000000 ) ) ;
#2165=VERTEX_POINT ( 'NONE', #8309 ) ;
#2169=DIRECTION ( 'NONE',  ( 0.000000000000000000, 0.000000000000000000, -1.000000000000000000 ) ) ;
#2170=CARTESIAN_POINT ( 'NONE',  ( 470.0000000000000000, -20.00000000000000000, 250.0000000000000000 ) ) ;
#2174=DIRECTION ( 'NONE',  ( -1.000000000000000000, 0.000000000000000000, 0.000000000000000000 ) ) ;
#2176=PLANE ( 'NONE',  #1754 ) ;
#2177=FACE_OUTER_BOUND ( 'NONE', #9843, .T. ) ;
#2179=DIRECTION ( 'NONE',  ( 1.000000000000000000, 0.000000000000000000, 0.000000000000000000 ) ) ;
#2180=FACE_OUTER_BOUND ( 'NONE', #10622, .T. ) ;
#2187=ORIENTED_EDGE ( 'NONE', *, *, #13580, .F. ) ;
#2191=CARTESIAN_POINT ( 'NONE',  ( 302.5000000000000000, -36.99999999999997868, -169.9999999999999716 ) ) ;
#2193=FACE_OUTER_BOUND ( 'NONE', #10787, .T. ) ;
#2201=ORIENTED_EDGE ( 'NONE', *, *, #5037, .T. ) ;
#2204=ORIENTED_EDGE ( 'NONE', *, *, #13849, .F. ) ;
#2205=CARTESIAN_POINT ( 'NONE',  ( 145.5000000000000284, -95.00000000000008527, -190.0000000000000000 ) ) ;
#2206=FACE_BOUND ( 'NONE', #10374, .T. ) ;
#2207=LINE ( 'NONE', #3316, #9921 ) ;
#2210=AXIS2_PLACEMENT_3D ( 'NONE', #5378, #9807, #6534 ) ;
#2212=DIRECTION ( 'NONE',  ( -0.000000000000000000, -0.000000000000000000, 1.000000000000000000 ) ) ;
#2215=VERTEX_POINT ( 'NONE', #4326 ) ;
#2224=EDGE_CURVE ( 'NONE', #12771, #8099, #3109, .T. ) ;
#2225=VECTOR ( 'NONE', #13991, 1000.000000000000000 ) ;
#2227=DIRECTION ( 'NONE',  ( 1.000000000000000000, 0.000000000000000000, 0.000000000000000000 ) ) ;
#2230=EDGE_CURVE ( 'NONE', #5572, #10689, #13888, .T. ) ;
#2234=AXIS2_PLACEMENT_3D ( 'NONE', #1608, #12858, #732 ) ;
#2241=EDGE_CURVE ( 'NONE', #3696, #7324, #4169, .T. ) ;
#2243=DIRECTION ( 'NONE',  ( -1.000000000000000000, 0.000000000000000000, -0.000000000000000000 ) ) ;
#2244=VECTOR ( 'NONE', #1390, 1000.000000000000000 ) ;
#2249=DIRECTION ( 'NONE',  ( -0.000000000000000000, 1.000000000000000000, -0.000000000000000000 ) ) ;
#2253=EDGE_CURVE ( 'NONE', #11549, #770, #1372, .T. ) ;
#2261=CYLINDRICAL_SURFACE ( 'NONE', #3990, 2.649999999999985700 ) ;
#2266=CARTESIAN_POINT ( 'NONE',  ( 319.9999999999999432, -225.0010000000000048, -19.99999999999998934 ) ) ;
#2270=DIRECTION ( 'NONE',  ( 0.000000000000000000, 0.000000000000000000, -1.000000000000000000 ) ) ;
#2277=AXIS2_PLACEMENT_3D ( 'NONE', #7218, #5990, #9334 ) ;
#2285=ORIENTED_EDGE ( 'NONE', *, *, #4791, .F. ) ;
#2291=ORIENTED_EDGE ( 'NONE', *, *, #13026, .F. ) ;
#2293=VECTOR ( 'NONE', #10382, 1000.000000000000000 ) ;
#2306=ORIENTED_EDGE ( 'NONE', *, *, #11640, .T. ) ;
#2312=DIRECTION ( 'NONE',  ( -0.000000000000000000, -0.000000000000000000, 1.000000000000000000 ) ) ;
#2316=AXIS2_PLACEMENT_3D ( 'NONE', #9483, #381, #12666 ) ;
#2318=AXIS2_PLACEMENT_3D ( 'NONE', #3055, #7467, #14038 ) ;
#2321=DIRECTION ( 'NONE',  ( -0.000000000000000000, -0.000000000000000000, -1.000000000000000000 ) ) ;
#2330=DIRECTION ( 'NONE',  ( -0.000000000000000000, -0.000000000000000000, -1.000000000000000000 ) ) ;
#2338=VERTEX_POINT ( 'NONE', #4611 ) ;
#2339=AXIS2_PLACEMENT_3D ( 'NONE', #541, #6227, #9420 ) ;
#2342=DIRECTION ( 'NONE',  ( -0.000000000000000000, -1.000000000000000000, -0.000000000000000000 ) ) ;
#2344=AXIS2_PLACEMENT_3D ( 'NONE', #13518, #3808, #3597 ) ;
#2345=CARTESIAN_POINT ( 'NONE',  ( 303.3333333333333144, -20.00000000000000000, 225.1500000000000625 ) ) ;
#2349=AXIS2_PLACEMENT_3D ( 'NONE', #4901, #7139, #10404 ) ;
#2352=DIRECTION ( 'NONE',  ( 0.000000000000000000, 1.000000000000000000, 0.000000000000000000 ) ) ;
#2353=AXIS2_PLACEMENT_3D ( 'NONE', #8008, #11506, #5993 ) ;
#2357=CARTESIAN_POINT ( 'NONE',  ( 140.0000000000000000, -75.00000000000008527, 169.9999999999999716 ) ) ;
#2365=VECTOR ( 'NONE', #2020, 1000.000000000000000 ) ;
#2372=VERTEX_POINT ( 'NONE', #10329 ) ;
#2375=EDGE_CURVE ( 'NONE', #9732, #1808, #1728, .T. ) ;
#2376=AXIS2_PLACEMENT_3D ( 'NONE', #4730, #2543, #262 ) ;
#2385=ORIENTED_EDGE ( 'NONE', *, *, #14034, .F. ) ;
#2387=CYLINDRICAL_SURFACE ( 'NONE', #13806, 2.500000000000002220 ) ;
#2391=LINE ( 'NONE', #12469, #1159 ) ;
#2402=LINE ( 'NONE', #9137, #4242 ) ;
#2411=DIRECTION ( 'NONE',  ( 0.000000000000000000, 0.000000000000000000, -1.000000000000000000 ) ) ;
#2423=CARTESIAN_POINT ( 'NONE',  ( 299.9999999999999432, -75.00000000000008527, -186.2999999999999829 ) ) ;
#2424=EDGE_CURVE ( 'NONE', #8882, #10563, #11943, .T. ) ;
#2430=DIRECTION ( 'NONE',  ( -1.000000000000000000, 0.000000000000000000, 0.000000000000000000 ) ) ;
#2431=EDGE_CURVE ( 'NONE', #770, #11549, #14243, .T. ) ;
#2432=ORIENTED_EDGE ( 'NONE', *, *, #878, .T. ) ;
#2444=ORIENTED_EDGE ( 'NONE', *, *, #2929, .T. ) ;
#2449=AXIS2_PLACEMENT_3D ( 'NONE', #4141, #989, #12044 ) ;
#2452=LINE ( 'NONE', #12178, #4315 ) ;
#2455=CARTESIAN_POINT ( 'NONE',  ( 136.6666666666666288, -20.00000000000000000, 219.8500000000001080 ) ) ;
#2463=ORIENTED_EDGE ( 'NONE', *, *, #11515, .T. ) ;
#2466=LINE ( 'NONE', #1442, #1966 ) ;
#2469=DIRECTION ( 'NONE',  ( 0.000000000000000000, 1.000000000000000000, 0.000000000000000000 ) ) ;
#2472=DIRECTION ( 'NONE',  ( -1.000000000000000000, 0.000000000000000000, 0.000000000000000000 ) ) ;
#2474=CONICAL_SURFACE ( 'NONE', #13125, 2.500000000000002220, 1.029744260000002631 ) ;
#2477=DIRECTION ( 'NONE',  ( -0.000000000000000000, -0.000000000000000000, -1.000000000000000000 ) ) ;
#2479=EDGE_CURVE ( 'NONE', #5504, #1662, #3149, .T. ) ;
#2489=ORIENTED_EDGE ( 'NONE', *, *, #4088, .F. ) ;
#2499=CARTESIAN_POINT ( 'NONE',  ( -30.00000000000002842, -225.0000000000000000, 169.9999999999999716 ) ) ;
#2506=LINE ( 'NONE', #11639, #8355 ) ;
#2519=FACE_OUTER_BOUND ( 'NONE', #4094, .T. ) ;
#2530=FACE_OUTER_BOUND ( 'NONE', #13466, .T. ) ;
#2534=DIRECTION ( 'NONE',  ( -0.000000000000000000, -0.000000000000000000, 1.000000000000000000 ) ) ;
#2535=LINE ( 'NONE', #5794, #9550 ) ;
#2543=DIRECTION ( 'NONE',  ( -0.000000000000000000, -0.000000000000000000, -1.000000000000000000 ) ) ;
#2544=VECTOR ( 'NONE', #7995, 1000.000000000000000 ) ;
#2559=CARTESIAN_POINT ( 'NONE',  ( 233.9999999999999432, -85.00000000000007105, 180.0000000000000000 ) ) ;
#2561=AXIS2_PLACEMENT_3D ( 'NONE', #4890, #10391, #19 ) ;
#2563=VERTEX_POINT ( 'NONE', #4593 ) ;
#2568=LINE ( 'NONE', #9382, #5482 ) ;
#2569=VERTEX_POINT ( 'NONE', #7842 ) ;
#2572=CIRCLE ( 'NONE', #10684, 2.500000000000002220 ) ;
#2576=CARTESIAN_POINT ( 'NONE',  ( 305.0000000000000000, -56.99999999999997158, -169.9999999999999716 ) ) ;
#2578=DIRECTION ( 'NONE',  ( -1.000000000000000000, 0.000000000000000000, 0.000000000000000000 ) ) ;
#2583=DIRECTION ( 'NONE',  ( -0.000000000000000000, -0.000000000000000000, 1.000000000000000000 ) ) ;
#2590=ADVANCED_FACE ( 'NONE', ( #7705 ), #4308, .F. ) ;
#2603=CARTESIAN_POINT ( 'NONE',  ( -30.00000000000002842, -25.00000000000000000, 250.0000000000000000 ) ) ;
#2605=CARTESIAN_POINT ( 'NONE',  ( 206.0000000000000284, -85.00000000000007105, 190.0000000000000000 ) ) ;
#2611=DIRECTION ( 'NONE',  ( 0.000000000000000000, 0.000000000000000000, 1.000000000000000000 ) ) ;
#2612=ORIENTED_EDGE ( 'NONE', *, *, #13192, .F. ) ;
#2616=EDGE_CURVE ( 'NONE', #13651, #6940, #10457, .T. ) ;
#2617=DIRECTION ( 'NONE',  ( -0.000000000000000000, 1.000000000000000000, -0.000000000000000000 ) ) ;
#2618=EDGE_LOOP ( 'NONE', ( #14249, #12035, #8287, #11770 ) ) ;
#2623=CARTESIAN_POINT ( 'NONE',  ( 319.9999999999999432, -24.99999999999999289, -169.9999999999999716 ) ) ;
#2627=CARTESIAN_POINT ( 'NONE',  ( 297.3499999999999659, -95.00000000000008527, 186.2999999999999829 ) ) ;
#2629=DIRECTION ( 'NONE',  ( -0.000000000000000000, -0.000000000000000000, 1.000000000000000000 ) ) ;
#2632=FACE_BOUND ( 'NONE', #1888, .T. ) ;
#2643=CARTESIAN_POINT ( 'NONE',  ( 303.3333333333333144, -20.00000000000000000, -225.1500000000000625 ) ) ;
#2650=DIRECTION ( 'NONE',  ( -0.000000000000000000, -0.000000000000000000, 1.000000000000000000 ) ) ;
#2651=CARTESIAN_POINT ( 'NONE',  ( 137.3500000000000227, -95.00000000000008527, -169.9999999999999716 ) ) ;
#2654=CYLINDRICAL_SURFACE ( 'NONE', #2353, 2.649999999999985700 ) ;
#2662=ORIENTED_EDGE ( 'NONE', *, *, #7023, .F. ) ;
#2663=FACE_OUTER_BOUND ( 'NONE', #1603, .T. ) ;
#2671=CARTESIAN_POINT ( 'NONE',  ( 137.3500000000000227, -95.00000000000008527, 190.0000000000000000 ) ) ;
#2672=EDGE_CURVE ( 'NONE', #2854, #6402, #2053, .T. ) ;
#2674=DIRECTION ( 'NONE',  ( -0.000000000000000000, -0.000000000000000000, 1.000000000000000000 ) ) ;
#2675=CARTESIAN_POINT ( 'NONE',  ( 203.5000000000000000, -85.00000000000007105, 190.0000000000000000 ) ) ;
#2681=AXIS2_PLACEMENT_3D ( 'NONE', #5396, #4305, #8657 ) ;
#2682=ORIENTED_EDGE ( 'NONE', *, *, #1154, .T. ) ;
#2684=DIRECTION ( 'NONE',  ( -0.000000000000000000, -0.000000000000000000, 1.000000000000000000 ) ) ;
#2689=DIRECTION ( 'NONE',  ( -1.000000000000000000, 0.000000000000000000, 0.000000000000000000 ) ) ;
#2691=ADVANCED_FACE ( 'NONE', ( #3640 ), #12349, .T. ) ;
#2694=ORIENTED_EDGE ( 'NONE', *, *, #9241, .T. ) ;
#2696=ADVANCED_FACE ( 'NONE', ( #9148 ), #3572, .F. ) ;
#2697=DIRECTION ( 'NONE',  ( -1.000000000000000000, 0.000000000000000000, 0.000000000000000000 ) ) ;
#2700=CARTESIAN_POINT ( 'NONE',  ( 219.9999999999999716, -85.00000000000007105, 190.0000000000000000 ) ) ;
#2705=AXIS2_PLACEMENT_3D ( 'NONE', #8929, #11660, #604 ) ;
#2706=EDGE_LOOP ( 'NONE', ( #9877, #11737, #6542, #7671 ) ) ;
#2716=FACE_BOUND ( 'NONE', #8671, .T. ) ;
#2719=DIRECTION ( 'NONE',  ( -0.000000000000000000, -0.000000000000000000, 1.000000000000000000 ) ) ;
#2721=CYLINDRICAL_SURFACE ( 'NONE', #2991, 2.649999999999985700 ) ;
#2724=AXIS2_PLACEMENT_3D ( 'NONE', #14154, #8655, #13869 ) ;
#2725=ORIENTED_EDGE ( 'NONE', *, *, #693, .F. ) ;
#2729=CARTESIAN_POINT ( 'NONE',  ( 119.9999999999999147, -20.00000000000000000, -19.99999999999998934 ) ) ;
#2731=CIRCLE ( 'NONE', #14297, 2.649999999999985700 ) ;
#2734=VECTOR ( 'NONE', #11680, 1000.000000000000000 ) ;
#2740=SHAPE_REPRESENTATION ( 'base table', ( #14039 ), #7000 ) ;
#2743=DIRECTION ( 'NONE',  ( -0.000000000000000000, -0.000000000000000000, 1.000000000000000000 ) ) ;
#2746=VERTEX_POINT ( 'NONE', #1665 ) ;
#2750=CARTESIAN_POINT ( 'NONE',  ( 134.9999999999999432, -36.99999999999997868, -169.9999999999999716 ) ) ;
#2752=CIRCLE ( 'NONE', #8074, 5.500000000000005329 ) ;
#2765=DIRECTION ( 'NONE',  ( 0.000000000000000000, 0.000000000000000000, -1.000000000000000000 ) ) ;
#2768=CARTESIAN_POINT ( 'NONE',  ( -30.00000000000002842, -25.00000000000000000, 250.0000000000000000 ) ) ;
#2769=DIRECTION ( 'NONE',  ( -1.000000000000000000, 0.000000000000000000, 0.000000000000000000 ) ) ;
#2771=DIRECTION ( 'NONE',  ( -1.000000000000000000, 0.000000000000000000, 0.000000000000000000 ) ) ;
#2773=EDGE_CURVE ( 'NONE', #1006, #1448, #8637, .T. ) ;
#2777=EDGE_CURVE ( 'NONE', #7324, #3696, #11882, .T. ) ;
#2785=DIRECTION ( 'NONE',  ( 0.000000000000000000, 0.000000000000000000, 1.000000000000000000 ) ) ;
#2792=VECTOR ( 'NONE', #10884, 1000.000000000000000 ) ;
#2797=ORIENTED_EDGE ( 'NONE', *, *, #9345, .F. ) ;
#2802=FACE_OUTER_BOUND ( 'NONE', #1531, .T. ) ;
#2811=CARTESIAN_POINT ( 'NONE',  ( 469.9999999999998863, -225.0000000000000000, -190.0000000000000000 ) ) ;
#2813=CONICAL_SURFACE ( 'NONE', #5584, 2.500000000000002220, 1.029744260000002631 ) ;
#2814=VERTEX_POINT ( 'NONE', #7260 ) ;
#2817=AXIS2_PLACEMENT_3D ( 'NONE', #1926, #8379, #11945 ) ;
#2824=FACE_OUTER_BOUND ( 'NONE', #13768, .T. ) ;
#2829=ORIENTED_EDGE ( 'NONE', *, *, #6117, .T. ) ;
#2834=CARTESIAN_POINT ( 'NONE',  ( 386.6666666666666288, -25.00000000000000000, 219.8500000000001080 ) ) ;
#2843=DIRECTION ( 'NONE',  ( -1.000000000000000000, 0.000000000000000000, 0.000000000000000000 ) ) ;
#2845=ORIENTED_EDGE ( 'NONE', *, *, #940, .T. ) ;
#2847=( GEOMETRIC_REPRESENTATION_CONTEXT ( 3 ) GLOBAL_UNCERTAINTY_ASSIGNED_CONTEXT ( ( #8575 ) ) GLOBAL_UNIT_ASSIGNED_CONTEXT ( ( #1091, #11261, #1205 ) ) REPRESENTATION_CONTEXT ( 'NONE', 'WORKASPACE' ) );
#2850=DIRECTION ( 'NONE',  ( 0.000000000000000000, 1.000000000000000000, 0.000000000000000000 ) ) ;
#2851=EDGE_CURVE ( 'NONE', #2569, #10145, #1676, .T. ) ;
#2854=VERTEX_POINT ( 'NONE', #641 ) ;
#2869=DIRECTION ( 'NONE',  ( -1.000000000000000000, 0.000000000000000000, 0.000000000000000000 ) ) ;
#2872=VERTEX_POINT ( 'NONE', #12699 ) ;
#2888=DIRECTION ( 'NONE',  ( -0.000000000000000000, 0.000000000000000000, 1.000000000000000000 ) ) ;
#2890=CARTESIAN_POINT ( 'NONE',  ( 229.9999999999999716, -85.00000000000007105, 169.9999999999999716 ) ) ;
#2891=ORIENTED_EDGE ( 'NONE', *, *, #7963, .T. ) ;
#2892=DIRECTION ( 'NONE',  ( -1.000000000000000000, 0.000000000000000000, 0.000000000000000000 ) ) ;
#2893=DIRECTION ( 'NONE',  ( -1.000000000000000000, 0.000000000000000000, 0.000000000000000000 ) ) ;
#2894=CYLINDRICAL_SURFACE ( 'NONE', #4649, 2.649999999999985700 ) ;
#2901=ORIENTED_EDGE ( 'NONE', *, *, #5908, .F. ) ;
#2902=CARTESIAN_POINT ( 'NONE',  ( 119.9999999999999147, -225.0010000000000048, 19.99999999999998934 ) ) ;
#2907=VERTEX_POINT ( 'NONE', #6677 ) ;
#2914=DIRECTION ( 'NONE',  ( -0.000000000000000000, -1.000000000000000000, -0.000000000000000000 ) ) ;
#2915=CYLINDRICAL_SURFACE ( 'NONE', #14123, 5.500000000000005329 ) ;
#2918=EDGE_CURVE ( 'NONE', #1381, #2563, #7751, .T. ) ;
#2920=VECTOR ( 'NONE', #7945, 1000.000000000000000 ) ;
#2924=VERTEX_POINT ( 'NONE', #11035 ) ;
#2926=ORIENTED_EDGE ( 'NONE', *, *, #12474, .T. ) ;
#2929=EDGE_CURVE ( 'NONE', #12902, #12884, #177, .T. ) ;
#2932=DIRECTION ( 'NONE',  ( -0.000000000000000000, -0.000000000000000000, -1.000000000000000000 ) ) ;
#2935=DIRECTION ( 'NONE',  ( 0.000000000000000000, 0.000000000000000000, -1.000000000000000000 ) ) ;
#2937=AXIS2_PLACEMENT_3D ( 'NONE', #7015, #13605, #9186 ) ;
#2941=CIRCLE ( 'NONE', #6174, 2.649999999999985700 ) ;
#2946=EDGE_CURVE ( 'NONE', #7986, #7291, #3916, .T. ) ;
#2947=DIRECTION ( 'NONE',  ( -0.000000000000000000, -0.000000000000000000, 1.000000000000000000 ) ) ;
#2948=ADVANCED_FACE ( 'NONE', ( #4364 ), #8706, .T. ) ;
#2958=CARTESIAN_POINT ( 'NONE',  ( -30.00000000000002842, -25.00000000000000000, -250.0000000000000000 ) ) ;
#2966=CIRCLE ( 'NONE', #8977, 10.00000000000000888 ) ;
#2969=ORIENTED_EDGE ( 'NONE', *, *, #4831, .T. ) ;
#2972=DIRECTION ( 'NONE',  ( 1.000000000000000000, 0.000000000000000000, 0.000000000000000000 ) ) ;
#2974=AXIS2_PLACEMENT_3D ( 'NONE', #10656, #4050, #6370 ) ;
#2991=AXIS2_PLACEMENT_3D ( 'NONE', #11641, #7140, #4028 ) ;
#2992=EDGE_CURVE ( 'NONE', #8157, #8189, #14213, .T. ) ;
#2993=DIRECTION ( 'NONE',  ( 0.000000000000000000, 0.000000000000000000, -1.000000000000000000 ) ) ;
#3001=ORIENTED_EDGE ( 'NONE', *, *, #13354, .F. ) ;
#3003=AXIS2_PLACEMENT_3D ( 'NONE', #9873, #1220, #5520 ) ;
#3008=CYLINDRICAL_SURFACE ( 'NONE', #12869, 2.500000000000002220 ) ;
#3013=CARTESIAN_POINT ( 'NONE',  ( 140.0000000000000000, -75.00000000000008527, -190.0000000000000000 ) ) ;
#3024=FACE_BOUND ( 'NONE', #6731, .T. ) ;
#3026=AXIS2_PLACEMENT_3D ( 'NONE', #2170, #6596, #1053 ) ;
#3027=CIRCLE ( 'NONE', #11354, 2.649999999999985700 ) ;
#3034=VERTEX_POINT ( 'NONE', #3354 ) ;
#3042=ADVANCED_FACE ( 'NONE', ( #6743, #11171, #5653, #3138, #7538, #11977 ), #918, .F. ) ;
#3049=EDGE_CURVE ( 'NONE', #11373, #8550, #8108, .T. ) ;
#3051=CARTESIAN_POINT ( 'NONE',  ( 53.33333333333330017, -20.00000000000000000, 222.5000000000000853 ) ) ;
#3055=CARTESIAN_POINT ( 'NONE',  ( 299.9999999999999432, -75.00000000000008527, -190.0000000000000000 ) ) ;
#3061=EDGE_CURVE ( 'NONE', #13280, #11549, #5719, .T. ) ;
#3063=ORIENTED_EDGE ( 'NONE', *, *, #9512, .T. ) ;
#3064=DIRECTION ( 'NONE',  ( -1.000000000000000000, 0.000000000000000000, 0.000000000000000000 ) ) ;
#3068=DIRECTION ( 'NONE',  ( 1.000000000000000000, 0.000000000000000000, 0.000000000000000000 ) ) ;
#3080=VECTOR ( 'NONE', #7090, 1000.000000000000000 ) ;
#3082=CARTESIAN_POINT ( 'NONE',  ( 305.0000000000000000, -36.99999999999997868, -169.9999999999999716 ) ) ;
#3083=ORIENTED_EDGE ( 'NONE', *, *, #8071, .T. ) ;
#3084=DIRECTION ( 'NONE',  ( 0.000000000000000000, 0.000000000000000000, -1.000000000000000000 ) ) ;
#3095=ORIENTED_EDGE ( 'NONE', *, *, #326, .T. ) ;
#3104=DIRECTION ( 'NONE',  ( 1.000000000000000000, 0.000000000000000000, 0.000000000000000000 ) ) ;
#3109=LINE ( 'NONE', #3178, #9962 ) ;
#3111=VERTEX_POINT ( 'NONE', #12542 ) ;
#3113=DIRECTION ( 'NONE',  ( 0.000000000000000000, 0.000000000000000000, -1.000000000000000000 ) ) ;
#3114=VERTEX_POINT ( 'NONE', #252 ) ;
#3125=VERTEX_POINT ( 'NONE', #8175 ) ;
#3132=ADVANCED_FACE ( 'NONE', ( #3692 ), #4719, .F. ) ;
#3135=AXIS2_PLACEMENT_3D ( 'NONE', #4151, #10977, #7621 ) ;
#3138=FACE_BOUND ( 'NONE', #10695, .T. ) ;
#3142=ORIENTED_EDGE ( 'NONE', *, *, #4024, .F. ) ;
#3143=EDGE_LOOP ( 'NONE', ( #4515, #1293, #3241, #7108, #5895, #1352, #3266, #6003 ) ) ;
#3149=CIRCLE ( 'NONE', #552, 2.649999999999985700 ) ;
#3151=EDGE_CURVE ( 'NONE', #2165, #11325, #1493, .T. ) ;
#3154=ORIENTED_EDGE ( 'NONE', *, *, #716, .F. ) ;
#3156=DIRECTION ( 'NONE',  ( -0.000000000000000000, -0.000000000000000000, 1.000000000000000000 ) ) ;
#3157=ORIENTED_EDGE ( 'NONE', *, *, #8229, .T. ) ;
#3158=CARTESIAN_POINT ( 'NONE',  ( 209.9999999999999716, -85.00000000000007105, -250.0009999999999764 ) ) ;
#3159=CARTESIAN_POINT ( 'NONE',  ( 319.9999999999999432, -25.00000000000000000, 169.9999999999999716 ) ) ;
#3162=FACE_OUTER_BOUND ( 'NONE', #9051, .T. ) ;
#3167=VERTEX_POINT ( 'NONE', #10077 ) ;
#3170=PLANE ( 'NONE',  #4834 ) ;
#3173=DIRECTION ( 'NONE',  ( 1.000000000000000000, 0.000000000000000000, 0.000000000000000000 ) ) ;
#3174=EDGE_CURVE ( 'NONE', #9742, #4689, #5798, .T. ) ;
#3178=CARTESIAN_POINT ( 'NONE',  ( 319.9999999999999432, -225.0010000000000048, -169.9999999999999716 ) ) ;
#3186=VECTOR ( 'NONE', #7303, 1000.000000000000000 ) ;
#3189=CIRCLE ( 'NONE', #12903, 2.649999999999985700 ) ;
#3194=AXIS2_PLACEMENT_3D ( 'NONE', #10986, #10911, #14094 ) ;
#3196=EDGE_CURVE ( 'NONE', #4280, #2907, #2391, .T. ) ;
#3198=CARTESIAN_POINT ( 'NONE',  ( 140.0000000000000000, -75.00000000000008527, -190.0000000000000000 ) ) ;
#3199=AXIS2_PLACEMENT_3D ( 'NONE', #12410, #2477, #10237 ) ;
#3200=EDGE_LOOP ( 'NONE', ( #9800, #5544 ) ) ;
#3203=ORIENTED_EDGE ( 'NONE', *, *, #1169, .F. ) ;
#3219=EDGE_CURVE ( 'NONE', #701, #11518, #13675, .T. ) ;
#3220=FACE_OUTER_BOUND ( 'NONE', #12586, .T. ) ;
#3224=VECTOR ( 'NONE', #4895, 1000.000000000000000 ) ;
#3228=FACE_BOUND ( 'NONE', #8580, .T. ) ;
#3231=CARTESIAN_POINT ( 'NONE',  ( 206.0000000000000284, -85.00000000000007105, 180.0000000000000000 ) ) ;
#3239=ORIENTED_EDGE ( 'NONE', *, *, #1614, .F. ) ;
#3241=ORIENTED_EDGE ( 'NONE', *, *, #3914, .T. ) ;
#3242=DIRECTION ( 'NONE',  ( -0.000000000000000000, -0.000000000000000000, -1.000000000000000000 ) ) ;
#3243=CARTESIAN_POINT ( 'NONE',  ( 137.4999999999999432, -56.99999999999997158, -180.0000000000000000 ) ) ;
#3244=DIRECTION ( 'NONE',  ( -0.000000000000000000, -0.000000000000000000, 1.000000000000000000 ) ) ;
#3247=EDGE_CURVE ( 'NONE', #3293, #4498, #11363, .T. ) ;
#3250=DIRECTION ( 'NONE',  ( -0.000000000000000000, -0.000000000000000000, -1.000000000000000000 ) ) ;
#3251=ADVANCED_FACE ( 'NONE', ( #2824 ), #2894, .F. ) ;
#3252=ORIENTED_EDGE ( 'NONE', *, *, #12759, .T. ) ;
#3253=ORIENTED_EDGE ( 'NONE', *, *, #4457, .F. ) ;
#3259=ORIENTED_EDGE ( 'NONE', *, *, #6973, .F. ) ;
#3260=CARTESIAN_POINT ( 'NONE',  ( 140.0000000000000000, -75.00000000000008527, 169.9999999999999716 ) ) ;
#3264=AXIS2_PLACEMENT_3D ( 'NONE', #721, #5113, #13866 ) ;
#3266=ORIENTED_EDGE ( 'NONE', *, *, #665, .F. ) ;
#3268=ORIENTED_EDGE ( 'NONE', *, *, #1868, .T. ) ;
#3270=CARTESIAN_POINT ( 'NONE',  ( 302.5000000000000000, -56.99999999999997158, -180.0000000000000000 ) ) ;
#3279=CARTESIAN_POINT ( 'NONE',  ( 119.9999999999999147, -24.99999999999999289, 169.9999999999999716 ) ) ;
#3285=AXIS2_PLACEMENT_3D ( 'NONE', #6219, #14044, #1934 ) ;
#3293=VERTEX_POINT ( 'NONE', #10659 ) ;
#3296=DIRECTION ( 'NONE',  ( -0.000000000000000000, -0.000000000000000000, 1.000000000000000000 ) ) ;
#3297=CYLINDRICAL_SURFACE ( 'NONE', #4577, 2.649999999999985700 ) ;
#3313=DIRECTION ( 'NONE',  ( 0.000000000000000000, 0.000000000000000000, 1.000000000000000000 ) ) ;
#3316=CARTESIAN_POINT ( 'NONE',  ( 469.9999999999998863, -225.0000000000000000, 169.9999999999999716 ) ) ;
#3317=VERTEX_POINT ( 'NONE', #6296 ) ;
#3318=EDGE_CURVE ( 'NONE', #13543, #6044, #7383, .T. ) ;
#3323=CARTESIAN_POINT ( 'NONE',  ( 219.9999999999999716, -20.00000000000000000, 225.1500000000000625 ) ) ;
#3334=DIRECTION ( 'NONE',  ( 0.000000000000000000, 0.000000000000000000, -1.000000000000000000 ) ) ;
#3336=CARTESIAN_POINT ( 'NONE',  ( 140.0000000000000000, -75.00000000000008527, 186.2999999999999829 ) ) ;
#3338=CARTESIAN_POINT ( 'NONE',  ( 140.0000000000000000, -75.00000000000008527, -190.0000000000000000 ) ) ;
#3340=LINE ( 'NONE', #13319, #6672 ) ;
#3344=VERTEX_POINT ( 'NONE', #10114 ) ;
#3347=EDGE_LOOP ( 'NONE', ( #4482, #14162 ) ) ;
#3354=CARTESIAN_POINT ( 'NONE',  ( 238.9999999999999432, -85.00000000000007105, 190.0000000000000000 ) ) ;
#3355=DIRECTION ( 'NONE',  ( -0.000000000000000000, 1.000000000000000000, -0.000000000000000000 ) ) ;
#3364=ORIENTED_EDGE ( 'NONE', *, *, #1687, .F. ) ;
#3365=CARTESIAN_POINT ( 'NONE',  ( 297.3499999999999659, -75.00000000000008527, 169.9999999999999716 ) ) ;
#3370=FACE_OUTER_BOUND ( 'NONE', #12461, .T. ) ;
#3377=VERTEX_POINT ( 'NONE', #4405 ) ;
#3381=DIRECTION ( 'NONE',  ( 0.000000000000000000, 0.000000000000000000, -1.000000000000000000 ) ) ;
#3391=CIRCLE ( 'NONE', #11486, 2.649999999999985700 ) ;
#3394=DIRECTION ( 'NONE',  ( -0.000000000000000000, -1.000000000000000000, -0.000000000000000000 ) ) ;
#3399=EDGE_CURVE ( 'NONE', #13571, #11552, #12, .T. ) ;
#3402=CARTESIAN_POINT ( 'NONE',  ( 140.0000000000000000, -95.00000000000008527, -186.2999999999999829 ) ) ;
#3410=ORIENTED_EDGE ( 'NONE', *, *, #12867, .F. ) ;
#3412=AXIS2_PLACEMENT_3D ( 'NONE', #4033, #11717, #5338 ) ;
#3428=ORIENTED_EDGE ( 'NONE', *, *, #7357, .F. ) ;
#3434=EDGE_CURVE ( 'NONE', #5319, #11916, #223, .T. ) ;
#3435=ORIENTED_EDGE ( 'NONE', *, *, #12521, .T. ) ;
#3444=LINE ( 'NONE', #1380, #9685 ) ;
#3451=CARTESIAN_POINT ( 'NONE',  ( 119.9999999999999147, -20.00000000000000000, 19.99999999999998934 ) ) ;
#3454=LINE ( 'NONE', #5627, #12535 ) ;
#3469=CARTESIAN_POINT ( 'NONE',  ( 294.4999999999999432, -75.00000000000008527, -186.2999999999999829 ) ) ;
#3471=ADVANCED_FACE ( 'NONE', ( #10550 ), #2813, .F. ) ;
#3473=ORIENTED_EDGE ( 'NONE', *, *, #947, .F. ) ;
#3477=EDGE_CURVE ( 'NONE', #4689, #9742, #10450, .T. ) ;
#3483=DIRECTION ( 'NONE',  ( 1.000000000000000000, 0.000000000000000000, 0.000000000000000000 ) ) ;
#3484=VECTOR ( 'NONE', #750, 1000.000000000000000 ) ;
#3486=DIRECTION ( 'NONE',  ( -0.000000000000000000, -0.000000000000000000, -1.000000000000000000 ) ) ;
#3488=DIRECTION ( 'NONE',  ( 0.000000000000000000, 0.000000000000000000, -1.000000000000000000 ) ) ;
#3493=DIRECTION ( 'NONE',  ( -0.000000000000000000, -0.000000000000000000, 1.000000000000000000 ) ) ;
#3496=AXIS2_PLACEMENT_3D ( 'NONE', #10250, #12495, #12634 ) ;
#3498=EDGE_CURVE ( 'NONE', #5927, #9740, #8599, .T. ) ;
#3500=ADVANCED_FACE ( 'NONE', ( #11563 ), #5905, .F. ) ;
#3501=CARTESIAN_POINT ( 'NONE',  ( 299.9999999999999432, -95.00000000000008527, -186.2999999999999829 ) ) ;
#3503=VECTOR ( 'NONE', #6008, 1000.000000000000000 ) ;
#3505=DIRECTION ( 'NONE',  ( 0.000000000000000000, 0.000000000000000000, 1.000000000000000000 ) ) ;
#3507=EDGE_CURVE ( 'NONE', #1452, #1662, #4970, .T. ) ;
#3510=VECTOR ( 'NONE', #12822, 1000.000000000000000 ) ;
#3513=ORIENTED_EDGE ( 'NONE', *, *, #12353, .F. ) ;
#3517=VECTOR ( 'NONE', #299, 1000.000000000000000 ) ;
#3518=ORIENTED_EDGE ( 'NONE', *, *, #4544, .F. ) ;
#3521=DIRECTION ( 'NONE',  ( -0.000000000000000000, 1.000000000000000000, -0.000000000000000000 ) ) ;
#3525=AXIS2_PLACEMENT_3D ( 'NONE', #10151, #1216, #9060 ) ;
#3547=ADVANCED_FACE ( 'NONE', ( #10261 ), #3730, .F. ) ;
#3558=ORIENTED_EDGE ( 'NONE', *, *, #1827, .F. ) ;
#3559=ORIENTED_EDGE ( 'NONE', *, *, #940, .F. ) ;
#3562=CARTESIAN_POINT ( 'NONE',  ( 119.9999999999999147, -225.0010000000000048, -19.99999999999998934 ) ) ;
#3563=EDGE_CURVE ( 'NONE', #2924, #11304, #5047, .T. ) ;
#3564=EDGE_CURVE ( 'NONE', #9136, #8882, #2506, .T. ) ;
#3565=ORIENTED_EDGE ( 'NONE', *, *, #1868, .F. ) ;
#3566=FACE_BOUND ( 'NONE', #13187, .T. ) ;
#3568=DIRECTION ( 'NONE',  ( 1.000000000000000000, 0.000000000000000000, 0.000000000000000000 ) ) ;
#3572=CYLINDRICAL_SURFACE ( 'NONE', #9498, 2.649999999999985700 ) ;
#3574=MANIFOLD_SOLID_BREP ( 'AdvancedHole2', #4054 ) ;
#3583=PLANE ( 'NONE',  #6507 ) ;
#3593=DIRECTION ( 'NONE',  ( 0.000000000000000000, 0.000000000000000000, 1.000000000000000000 ) ) ;
#3594=VERTEX_POINT ( 'NONE', #12801 ) ;
#3597=DIRECTION ( 'NONE',  ( -1.000000000000000000, 0.000000000000000000, 0.000000000000000000 ) ) ;
#3599=DIRECTION ( 'NONE',  ( 0.000000000000000000, 0.000000000000000000, -1.000000000000000000 ) ) ;
#3600=ADVANCED_FACE ( 'NONE', ( #14015 ), #10845, .F. ) ;
#3603=AXIS2_PLACEMENT_3D ( 'NONE', #2266, #2157, #11125 ) ;
#3610=AXIS2_PLACEMENT_3D ( 'NONE', #4855, #11445, #8024 ) ;
#3617=DIRECTION ( 'NONE',  ( -0.000000000000000000, -0.000000000000000000, -1.000000000000000000 ) ) ;
#3626=ORIENTED_EDGE ( 'NONE', *, *, #14034, .T. ) ;
#3629=ORIENTED_EDGE ( 'NONE', *, *, #1415, .T. ) ;
#3637=EDGE_LOOP ( 'NONE', ( #2187, #8085 ) ) ;
#3638=CARTESIAN_POINT ( 'NONE',  ( 119.9999999999999147, -25.00000000000000000, 169.9999999999999716 ) ) ;
#3640=FACE_OUTER_BOUND ( 'NONE', #6859, .T. ) ;
#3649=ORIENTED_EDGE ( 'NONE', *, *, #11650, .T. ) ;
#3652=VECTOR ( 'NONE', #13453, 1000.000000000000000 ) ;
#3660=CYLINDRICAL_SURFACE ( 'NONE', #11736, 2.649999999999985700 ) ;
#3661=AXIS2_PLACEMENT_3D ( 'NONE', #11522, #9491, #12825 ) ;
#3670=DIRECTION ( 'NONE',  ( -0.000000000000000000, -0.000000000000000000, 1.000000000000000000 ) ) ;
#3673=EDGE_CURVE ( 'NONE', #11569, #5871, #4671, .T. ) ;
#3674=VECTOR ( 'NONE', #7788, 1000.000000000000000 ) ;
#3684=CARTESIAN_POINT ( 'NONE',  ( 137.4999999999999432, -56.99999999999997158, -169.9999999999999716 ) ) ;
#3689=ORIENTED_EDGE ( 'NONE', *, *, #1610, .T. ) ;
#3690=CARTESIAN_POINT ( 'NONE',  ( 386.6666666666666288, -20.00000000000000000, -219.8500000000001080 ) ) ;
#3692=FACE_OUTER_BOUND ( 'NONE', #7470, .T. ) ;
#3696=VERTEX_POINT ( 'NONE', #6625 ) ;
#3699=CARTESIAN_POINT ( 'NONE',  ( 119.9999999999999147, -20.00000000000000000, -169.9999999999999716 ) ) ;
#3701=DIRECTION ( 'NONE',  ( 0.000000000000000000, 0.000000000000000000, 1.000000000000000000 ) ) ;
#3709=CARTESIAN_POINT ( 'NONE',  ( 319.9999999999999432, -20.00000000000000000, 19.99999999999998934 ) ) ;
#3710=ORIENTED_EDGE ( 'NONE', *, *, #3219, .T. ) ;
#3711=CIRCLE ( 'NONE', #11135, 10.00000000000000888 ) ;
#3713=CARTESIAN_POINT ( 'NONE',  ( 140.0000000000000000, -95.00000000000008527, 186.2999999999999829 ) ) ;
#3718=ORIENTED_EDGE ( 'NONE', *, *, #5882, .T. ) ;
#3719=DIRECTION ( 'NONE',  ( 1.000000000000000000, 0.000000000000000000, 0.000000000000000000 ) ) ;
#3720=VERTEX_POINT ( 'NONE', #2345 ) ;
#3728=CARTESIAN_POINT ( 'NONE',  ( 386.6666666666666288, -25.00000000000000000, 222.5000000000000853 ) ) ;
#3730=CYLINDRICAL_SURFACE ( 'NONE', #6968, 5.500000000000005329 ) ;
#3733=EDGE_CURVE ( 'NONE', #1448, #1006, #3027, .T. ) ;
#3770=DIRECTION ( 'NONE',  ( 1.000000000000000000, 0.000000000000000000, 0.000000000000000000 ) ) ;
#3774=VERTEX_POINT ( 'NONE', #6031 ) ;
#3781=CARTESIAN_POINT ( 'NONE',  ( 302.6499999999999204, -95.00000000000008527, -186.2999999999999829 ) ) ;
#3783=DIRECTION ( 'NONE',  ( -0.000000000000000000, 1.000000000000000000, -0.000000000000000000 ) ) ;
#3790=DIRECTION ( 'NONE',  ( -1.000000000000000000, 0.000000000000000000, 0.000000000000000000 ) ) ;
#3795=DIRECTION ( 'NONE',  ( 1.000000000000000000, 0.000000000000000000, -0.000000000000000000 ) ) ;
#3805=ORIENTED_EDGE ( 'NONE', *, *, #3399, .F. ) ;
#3808=DIRECTION ( 'NONE',  ( -0.000000000000000000, -0.000000000000000000, 1.000000000000000000 ) ) ;
#3811=LINE ( 'NONE', #6425, #4363 ) ;
#3814=DIRECTION ( 'NONE',  ( 0.000000000000000000, 1.000000000000000000, 0.000000000000000000 ) ) ;
#3816=CARTESIAN_POINT ( 'NONE',  ( 119.9999999999999147, -24.99999999999999289, -19.99999999999998934 ) ) ;
#3817=EDGE_CURVE ( 'NONE', #11952, #10315, #3711, .T. ) ;
#3822=CARTESIAN_POINT ( 'NONE',  ( 299.9999999999999432, -95.00000000000008527, -190.0000000000000000 ) ) ;
#3833=LINE ( 'NONE', #7029, #5605 ) ;
#3842=ORIENTED_EDGE ( 'NONE', *, *, #3318, .F. ) ;
#3848=EDGE_CURVE ( 'NONE', #1662, #5504, #8130, .T. ) ;
#3856=AXIS2_PLACEMENT_3D ( 'NONE', #6707, #1181, #6569 ) ;
#3857=DIRECTION ( 'NONE',  ( 1.000000000000000000, 0.000000000000000000, 0.000000000000000000 ) ) ;
#3869=DIRECTION ( 'NONE',  ( -1.000000000000000000, 0.000000000000000000, 0.000000000000000000 ) ) ;
#3872=FACE_OUTER_BOUND ( 'NONE', #6127, .T. ) ;
#3876=DIRECTION ( 'NONE',  ( -0.000000000000000000, -0.000000000000000000, -1.000000000000000000 ) ) ;
#3878=ORIENTED_EDGE ( 'NONE', *, *, #5281, .T. ) ;
#3890=ORIENTED_EDGE ( 'NONE', *, *, #5593, .T. ) ;
#3891=EDGE_CURVE ( 'NONE', #8759, #8867, #10221, .T. ) ;
#3900=DIRECTION ( 'NONE',  ( -0.000000000000000000, -1.000000000000000000, -0.000000000000000000 ) ) ;
#3904=ADVANCED_FACE ( 'NONE', ( #11688 ), #12777, .F. ) ;
#3914=EDGE_CURVE ( 'NONE', #7589, #12061, #9591, .T. ) ;
#3916=CIRCLE ( 'NONE', #10874, 2.649999999999985700 ) ;
#3918=DIRECTION ( 'NONE',  ( -0.000000000000000000, -0.000000000000000000, -1.000000000000000000 ) ) ;
#3937=ADVANCED_FACE ( 'NONE', ( #6247 ), #2915, .F. ) ;
#3945=ORIENTED_EDGE ( 'NONE', *, *, #1947, .T. ) ;
#3948=CARTESIAN_POINT ( 'NONE',  ( 145.5000000000000284, -75.00000000000008527, -186.2999999999999829 ) ) ;
#3961=ORIENTED_EDGE ( 'NONE', *, *, #1323, .T. ) ;
#3962=VECTOR ( 'NONE', #7209, 1000.000000000000000 ) ;
#3969=AXIS2_PLACEMENT_3D ( 'NONE', #6325, #5314, #5024 ) ;
#3971=DIRECTION ( 'NONE',  ( -1.000000000000000000, 0.000000000000000000, 0.000000000000000000 ) ) ;
#3989=EDGE_LOOP ( 'NONE', ( #9097, #319, #9195, #6339 ) ) ;
#3990=AXIS2_PLACEMENT_3D ( 'NONE', #9744, #5389, #10903 ) ;
#3996=FACE_OUTER_BOUND ( 'NONE', #4248, .T. ) ;
#3998=ORIENTED_EDGE ( 'NONE', *, *, #11443, .T. ) ;
#3999=CARTESIAN_POINT ( 'NONE',  ( 302.5000000000000000, -36.99999999999997868, -169.9999999999999716 ) ) ;
#4007=VERTEX_POINT ( 'NONE', #10895 ) ;
#4009=ORIENTED_EDGE ( 'NONE', *, *, #3498, .T. ) ;
#4018=DIRECTION ( 'NONE',  ( -0.000000000000000000, -0.000000000000000000, 1.000000000000000000 ) ) ;
#4019=ORIENTED_EDGE ( 'NONE', *, *, #5003, .T. ) ;
#4021=UNCERTAINTY_MEASURE_WITH_UNIT (LENGTH_MEASURE( 1.000000000000000082E-05 ), #13661, 'distance_accuracy_value', 'NONE');
#4024=EDGE_CURVE ( 'NONE', #13843, #2907, #5760, .T. ) ;
#4026=CARTESIAN_POINT ( 'NONE',  ( 299.9999999999999432, -75.00000000000008527, 190.0000000000000000 ) ) ;
#4028=DIRECTION ( 'NONE',  ( -1.000000000000000000, 0.000000000000000000, 0.000000000000000000 ) ) ;
#4029=EDGE_LOOP ( 'NONE', ( #2489, #1510, #14104, #7830 ) ) ;
#4032=ORIENTED_EDGE ( 'NONE', *, *, #3891, .T. ) ;
#4033=CARTESIAN_POINT ( 'NONE',  ( 53.33333333333330017, -20.00000000000000000, -222.5000000000000853 ) ) ;
#4038=CARTESIAN_POINT ( 'NONE',  ( 137.3500000000000227, -95.00000000000008527, -190.0000000000000000 ) ) ;
#4048=ORIENTED_EDGE ( 'NONE', *, *, #6797, .T. ) ;
#4049=CARTESIAN_POINT ( 'NONE',  ( 136.6666666666666288, -20.00000000000000000, 222.5000000000000853 ) ) ;
#4050=DIRECTION ( 'NONE',  ( -0.000000000000000000, -0.000000000000000000, 1.000000000000000000 ) ) ;
#4054=CLOSED_SHELL ( 'NONE', ( #11214, #4234, #8536, #7391, #7168, #7433, #11817, #3500, #9860, #8351, #4533, #13486, #5300, #8802, #1986, #6586, #10847, #7541, #13769, #1935, #7769, #6143, #5670, #3471, #3904, #4281, #10217, #9177, #383, #12001, #12659, #4881, #4852, #11918, #3251, #13760, #7110, #2696, #4147, #5633, #6429, #3042, #7531, #1983, #2691, #7940, #14138, #9609, #9070, #5079, #7651, #684, #8766, #6108, #5430, #7084, #4633, #8429, #13205, #11004, #7961, #13240, #86, #639, #2948, #12709, #6924, #1711, #12673, #1193, #8976, #6231, #8584, #8877, #11801, #1168, #4906, #3600, #1173, #3937, #7646, #10387, #3132, #1460, #12716, #3547, #9138, #446, #6223, #11729, #4518, #9240, #6831, #5775, #950, #244, #6754, #4563, #1478, #11450, #9151, #2590, #5673, #7898, #6844, #8788 ) ) ;
#4067=ORIENTED_EDGE ( 'NONE', *, *, #7259, .F. ) ;
#4068=DIRECTION ( 'NONE',  ( -0.000000000000000000, -0.000000000000000000, -1.000000000000000000 ) ) ;
#4069=EDGE_CURVE ( 'NONE', #6338, #12042, #10405, .T. ) ;
#4074=CIRCLE ( 'NONE', #2681, 2.649999999999985700 ) ;
#4075=ORIENTED_EDGE ( 'NONE', *, *, #13590, .T. ) ;
#4076=ORIENTED_EDGE ( 'NONE', *, *, #8041, .F. ) ;
#4079=DIRECTION ( 'NONE',  ( 1.000000000000000000, 0.000000000000000000, 0.000000000000000000 ) ) ;
#4080=ORIENTED_EDGE ( 'NONE', *, *, #7815, .F. ) ;
#4088=EDGE_CURVE ( 'NONE', #2372, #12902, #5657, .T. ) ;
#4093=AXIS2_PLACEMENT_3D ( 'NONE', #4929, #8102, #2893 ) ;
#4094=EDGE_LOOP ( 'NONE', ( #10916, #7696, #8497, #8219 ) ) ;
#4095=CONICAL_SURFACE ( 'NONE', #12890, 2.500000000000002220, 1.029744260000002631 ) ;
#4104=AXIS2_PLACEMENT_3D ( 'NONE', #2750, #2674, #12394 ) ;
#4108=CARTESIAN_POINT ( 'NONE',  ( 305.0000000000000000, -56.99999999999997158, -180.0000000000000000 ) ) ;
#4112=CIRCLE ( 'NONE', #8508, 5.500000000000005329 ) ;
#4113=LINE ( 'NONE', #12739, #11816 ) ;
#4114=VERTEX_POINT ( 'NONE', #255 ) ;
#4115=AXIS2_PLACEMENT_3D ( 'NONE', #8199, #4957, #10613 ) ;
#4128=DIRECTION ( 'NONE',  ( -1.000000000000000000, 0.000000000000000000, 0.000000000000000000 ) ) ;
#4130=CONICAL_SURFACE ( 'NONE', #2974, 2.500000000000002220, 1.029744260000002631 ) ;
#4141=CARTESIAN_POINT ( 'NONE',  ( 305.0000000000000000, -36.99999999999997868, -169.9999999999999716 ) ) ;
#4144=PLANE ( 'NONE',  #11075 ) ;
#4147=ADVANCED_FACE ( 'NONE', ( #11526 ), #4936, .F. ) ;
#4151=CARTESIAN_POINT ( 'NONE',  ( 0.000000000000000000, -225.0000000000000000, 0.000000000000000000 ) ) ;
#4157=ORIENTED_EDGE ( 'NONE', *, *, #266, .F. ) ;
#4169=CIRCLE ( 'NONE', #5334, 2.649999999999985700 ) ;
#4170=EDGE_LOOP ( 'NONE', ( #5892, #3998, #5411, #14236 ) ) ;
#4174=VERTEX_POINT ( 'NONE', #8249 ) ;
#4175=FACE_OUTER_BOUND ( 'NONE', #11152, .T. ) ;
#4176=AXIS2_PLACEMENT_3D ( 'NONE', #7510, #6278, #10497 ) ;
#4178=DIRECTION ( 'NONE',  ( -0.000000000000000000, -0.000000000000000000, 1.000000000000000000 ) ) ;
#4179=CIRCLE ( 'NONE', #11582, 2.649999999999985700 ) ;
#4182=VECTOR ( 'NONE', #3068, 1000.000000000000000 ) ;
#4189=CIRCLE ( 'NONE', #11140, 2.500000000000002220 ) ;
#4196=LINE ( 'NONE', #6288, #3186 ) ;
#4197=AXIS2_PLACEMENT_3D ( 'NONE', #826, #3113, #7376 ) ;
#4207=VECTOR ( 'NONE', #10788, 1000.000000000000000 ) ;
#4209=CARTESIAN_POINT ( 'NONE',  ( 303.3333333333333144, -20.00000000000000000, 225.1500000000000625 ) ) ;
#4212=ORIENTED_EDGE ( 'NONE', *, *, #13180, .F. ) ;
#4214=ORIENTED_EDGE ( 'NONE', *, *, #3507, .T. ) ;
#4217=ORIENTED_EDGE ( 'NONE', *, *, #6336, .F. ) ;
#4219=DIRECTION ( 'NONE',  ( 0.000000000000000000, 0.000000000000000000, 1.000000000000000000 ) ) ;
#4221=AXIS2_PLACEMENT_3D ( 'NONE', #1349, #5786, #13396 ) ;
#4224=DIRECTION ( 'NONE',  ( -0.000000000000000000, 0.000000000000000000, 1.000000000000000000 ) ) ;
#4226=ORIENTED_EDGE ( 'NONE', *, *, #693, .T. ) ;
#4232=ORIENTED_EDGE ( 'NONE', *, *, #504, .T. ) ;
#4234=ADVANCED_FACE ( 'NONE', ( #9282 ), #6884, .F. ) ;
#4242=VECTOR ( 'NONE', #7037, 1000.000000000000000 ) ;
#4247=ORIENTED_EDGE ( 'NONE', *, *, #9968, .F. ) ;
#4248=EDGE_LOOP ( 'NONE', ( #3513, #677, #474, #11762 ) ) ;
#4249=PRODUCT_DEFINITION_FORMATION_WITH_SPECIFIED_SOURCE ( 'ANY', '', #173, .NOT_KNOWN. ) ;
#4251=EDGE_LOOP ( 'NONE', ( #6690, #2662 ) ) ;
#4255=PLANE ( 'NONE',  #12459 ) ;
#4273=DIRECTION ( 'NONE',  ( -0.000000000000000000, 1.000000000000000000, -0.000000000000000000 ) ) ;
#4275=DIRECTION ( 'NONE',  ( -0.000000000000000000, 1.000000000000000000, -0.000000000000000000 ) ) ;
#4280=VERTEX_POINT ( 'NONE', #1721 ) ;
#4281=ADVANCED_FACE ( 'NONE', ( #624 ), #10163, .F. ) ;
#4288=DIRECTION ( 'NONE',  ( -0.000000000000000000, 1.000000000000000000, -0.000000000000000000 ) ) ;
#4296=AXIS2_PLACEMENT_3D ( 'NONE', #9579, #7035, #11458 ) ;
#4299=DIRECTION ( 'NONE',  ( -0.000000000000000000, -0.000000000000000000, -1.000000000000000000 ) ) ;
#4301=EDGE_CURVE ( 'NONE', #13571, #3125, #2752, .T. ) ;
#4303=CARTESIAN_POINT ( 'NONE',  ( 299.9999999999999432, -95.00000000000008527, 190.0000000000000000 ) ) ;
#4304=ORIENTED_EDGE ( 'NONE', *, *, #12094, .F. ) ;
#4305=DIRECTION ( 'NONE',  ( -0.000000000000000000, 1.000000000000000000, -0.000000000000000000 ) ) ;
#4308=CYLINDRICAL_SURFACE ( 'NONE', #8544, 10.00000000000000888 ) ;
#4309=AXIS2_PLACEMENT_3D ( 'NONE', #9075, #1373, #3568 ) ;
#4315=VECTOR ( 'NONE', #11236, 1000.000000000000000 ) ;
#4319=FACE_BOUND ( 'NONE', #1172, .T. ) ;
#4321=VECTOR ( 'NONE', #8310, 1000.000000000000000 ) ;
#4324=CARTESIAN_POINT ( 'NONE',  ( 136.6666666666666288, -20.00000000000000000, 225.1500000000000625 ) ) ;
#4326=CARTESIAN_POINT ( 'NONE',  ( 470.0000000000000000, -20.00000000000000000, -250.0000000000000000 ) ) ;
#4329=EDGE_LOOP ( 'NONE', ( #9699, #789, #2969, #7377 ) ) ;
#4339=CIRCLE ( 'NONE', #6872, 5.500000000000005329 ) ;
#4341=PLANE ( 'NONE',  #5551 ) ;
#4361=DIRECTION ( 'NONE',  ( 0.000000000000000000, 0.000000000000000000, -1.000000000000000000 ) ) ;
#4363=VECTOR ( 'NONE', #8597, 1000.000000000000000 ) ;
#4364=FACE_OUTER_BOUND ( 'NONE', #10291, .T. ) ;
#4366=LINE ( 'NONE', #7753, #582 ) ;
#4370=EDGE_LOOP ( 'NONE', ( #6334, #6427, #330 ) ) ;
#4374=CARTESIAN_POINT ( 'NONE',  ( 136.6666666666666288, -20.00000000000000000, -222.5000000000000853 ) ) ;
#4384=CARTESIAN_POINT ( 'NONE',  ( 302.6499999999999204, -75.00000000000008527, 190.0000000000000000 ) ) ;
#4393=AXIS2_PLACEMENT_3D ( 'NONE', #8783, #6746, #11176 ) ;
#4394=ORIENTED_EDGE ( 'NONE', *, *, #7895, .F. ) ;
#4404=AXIS2_PLACEMENT_3D ( 'NONE', #1306, #4665, #11405 ) ;
#4405=CARTESIAN_POINT ( 'NONE',  ( 319.9999999999999432, -20.00000000000000000, 19.99999999999998934 ) ) ;
#4407=DIRECTION ( 'NONE',  ( -0.000000000000000000, 1.000000000000000000, -0.000000000000000000 ) ) ;
#4411=VECTOR ( 'NONE', #11096, 1000.000000000000000 ) ;
#4414=EDGE_CURVE ( 'NONE', #11304, #3344, #761, .T. ) ;
#4415=ORIENTED_EDGE ( 'NONE', *, *, #7815, .T. ) ;
#4423=DIRECTION ( 'NONE',  ( 1.000000000000000000, 0.000000000000000000, 0.000000000000000000 ) ) ;
#4427=VECTOR ( 'NONE', #3670, 1000.000000000000000 ) ;
#4428=ORIENTED_EDGE ( 'NONE', *, *, #9314, .T. ) ;
#4429=VERTEX_POINT ( 'NONE', #835 ) ;
#4435=CARTESIAN_POINT ( 'NONE',  ( 134.5000000000000000, -75.00000000000008527, 190.0000000000000000 ) ) ;
#4443=CARTESIAN_POINT ( 'NONE',  ( 219.9999999999999716, -20.00000000000000000, 219.8500000000001080 ) ) ;
#4444=ORIENTED_EDGE ( 'NONE', *, *, #164, .F. ) ;
#4450=DIRECTION ( 'NONE',  ( -0.000000000000000000, -0.000000000000000000, 1.000000000000000000 ) ) ;
#4454=PRESENTATION_STYLE_ASSIGNMENT (( #13967 ) ) ;
#4457=EDGE_CURVE ( 'NONE', #2121, #5322, #10649, .T. ) ;
#4458=CARTESIAN_POINT ( 'NONE',  ( 119.9999999999999147, -25.00000000000000000, -169.9999999999999716 ) ) ;
#4465=ORIENTED_EDGE ( 'NONE', *, *, #11034, .T. ) ;
#4467=VECTOR ( 'NONE', #6821, 1000.000000000000000 ) ;
#4468=LINE ( 'NONE', #7853, #2244 ) ;
#4478=CARTESIAN_POINT ( 'NONE',  ( -30.00000000000002842, -25.00000000000000000, -190.0000000000000000 ) ) ;
#4482=ORIENTED_EDGE ( 'NONE', *, *, #12474, .F. ) ;
#4485=CARTESIAN_POINT ( 'NONE',  ( 145.5000000000000284, -75.00000000000008527, -190.0000000000000000 ) ) ;
#4487=ORIENTED_EDGE ( 'NONE', *, *, #12241, .T. ) ;
#4498=VERTEX_POINT ( 'NONE', #3469 ) ;
#4505=DIRECTION ( 'NONE',  ( -1.000000000000000000, 0.000000000000000000, 0.000000000000000000 ) ) ;
#4508=CYLINDRICAL_SURFACE ( 'NONE', #2705, 2.649999999999985700 ) ;
#4515=ORIENTED_EDGE ( 'NONE', *, *, #8041, .T. ) ;
#4518=ADVANCED_FACE ( 'NONE', ( #6658, #1199 ), #4341, .F. ) ;
#4525=DIRECTION ( 'NONE',  ( 0.000000000000000000, 1.000000000000000000, 0.000000000000000000 ) ) ;
#4526=CIRCLE ( 'NONE', #1727, 2.500000000000002220 ) ;
#4532=LINE ( 'NONE', #3451, #13807 ) ;
#4533=ADVANCED_FACE ( 'NONE', ( #13257 ), #9925, .F. ) ;
#4534=PLANE ( 'NONE',  #1769 ) ;
#4542=ORIENTED_EDGE ( 'NONE', *, *, #2616, .F. ) ;
#4544=EDGE_CURVE ( 'NONE', #12208, #4429, #7624, .T. ) ;
#4561=ORIENTED_EDGE ( 'NONE', *, *, #7513, .F. ) ;
#4562=CARTESIAN_POINT ( 'NONE',  ( 142.6500000000000057, -75.00000000000008527, -186.2999999999999829 ) ) ;
#4563=ADVANCED_FACE ( 'NONE', ( #6800 ), #11225, .F. ) ;
#4564=VECTOR ( 'NONE', #3156, 1000.000000000000000 ) ;
#4569=DIRECTION ( 'NONE',  ( 0.000000000000000000, -0.000000000000000000, -1.000000000000000000 ) ) ;
#4570=CARTESIAN_POINT ( 'NONE',  ( 140.0000000000000000, -95.00000000000008527, -186.2999999999999829 ) ) ;
#4576=AXIS2_PLACEMENT_3D ( 'NONE', #3082, #4018, #10837 ) ;
#4577=AXIS2_PLACEMENT_3D ( 'NONE', #1012, #5668, #3505 ) ;
#4580=CYLINDRICAL_SURFACE ( 'NONE', #9387, 2.500000000000002220 ) ;
#4584=VECTOR ( 'NONE', #4288, 1000.000000000000000 ) ;
#4588=DIRECTION ( 'NONE',  ( 0.000000000000000000, 0.000000000000000000, -1.000000000000000000 ) ) ;
#4589=AXIS2_PLACEMENT_3D ( 'NONE', #5809, #10234, #5736 ) ;
#4590=CYLINDRICAL_SURFACE ( 'NONE', #10841, 2.649999999999985700 ) ;
#4592=EDGE_CURVE ( 'NONE', #6044, #8157, #7664, .T. ) ;
#4593=CARTESIAN_POINT ( 'NONE',  ( 386.6666666666666288, -20.00000000000000000, 225.1500000000000625 ) ) ;
#4597=ORIENTED_EDGE ( 'NONE', *, *, #4642, .T. ) ;
#4598=AXIS2_PLACEMENT_3D ( 'NONE', #12874, #4178, #3104 ) ;
#4602=VERTEX_POINT ( 'NONE', #13524 ) ;
#4611=CARTESIAN_POINT ( 'NONE',  ( 136.6666666666666288, -25.00000000000000000, 225.1500000000000625 ) ) ;
#4618=CIRCLE ( 'NONE', #1596, 2.649999999999985700 ) ;
#4619=CARTESIAN_POINT ( 'NONE',  ( -30.00000000000002842, -225.0000000000000000, -190.0000000000000000 ) ) ;
#4625=AXIS2_PLACEMENT_3D ( 'NONE', #10263, #290, #1541 ) ;
#4631=LINE ( 'NONE', #10140, #4411 ) ;
#4633=ADVANCED_FACE ( 'NONE', ( #2519 ), #12523, .F. ) ;
#4637=DIRECTION ( 'NONE',  ( -0.000000000000000000, -0.000000000000000000, 1.000000000000000000 ) ) ;
#4642=EDGE_CURVE ( 'NONE', #2814, #3317, #4618, .T. ) ;
#4645=CARTESIAN_POINT ( 'NONE',  ( 140.0000000000000000, -95.00000000000008527, -190.0000000000000000 ) ) ;
#4649=AXIS2_PLACEMENT_3D ( 'NONE', #4930, #9354, #13833 ) ;
#4655=CONICAL_SURFACE ( 'NONE', #4221, 2.500000000000002220, 1.029744260000002631 ) ;
#4665=DIRECTION ( 'NONE',  ( -1.000000000000000000, 0.000000000000000000, 0.000000000000000000 ) ) ;
#4666=AXIS2_PLACEMENT_3D ( 'NONE', #1260, #1333, #5696 ) ;
#4671=CIRCLE ( 'NONE', #12768, 2.500000000000002220 ) ;
#4673=ORIENTED_EDGE ( 'NONE', *, *, #6797, .F. ) ;
#4677=ORIENTED_EDGE ( 'NONE', *, *, #5239, .F. ) ;
#4679=EDGE_LOOP ( 'NONE', ( #13143, #1992, #5190 ) ) ;
#4680=DIRECTION ( 'NONE',  ( 0.000000000000000000, -0.000000000000000000, 1.000000000000000000 ) ) ;
#4689=VERTEX_POINT ( 'NONE', #11578 ) ;
#4693=DIRECTION ( 'NONE',  ( 1.000000000000000000, 0.000000000000000000, 0.000000000000000000 ) ) ;
#4697=ORIENTED_EDGE ( 'NONE', *, *, #13243, .T. ) ;
#4707=AXIS2_PLACEMENT_3D ( 'NONE', #11910, #2914, #13995 ) ;
#4711=ORIENTED_EDGE ( 'NONE', *, *, #1343, .T. ) ;
#4713=ORIENTED_EDGE ( 'NONE', *, *, #7204, .F. ) ;
#4715=DIRECTION ( 'NONE',  ( 0.000000000000000000, -0.000000000000000000, 1.000000000000000000 ) ) ;
#4719=CYLINDRICAL_SURFACE ( 'NONE', #7653, 5.500000000000005329 ) ;
#4727=LINE ( 'NONE', #1291, #5452 ) ;
#4730=CARTESIAN_POINT ( 'NONE',  ( 299.9999999999999432, -75.00000000000008527, -190.0000000000000000 ) ) ;
#4736=ORIENTED_EDGE ( 'NONE', *, *, #11567, .T. ) ;
#4741=EDGE_LOOP ( 'NONE', ( #1210, #14306, #6014, #8045 ) ) ;
#4742=ORIENTED_EDGE ( 'NONE', *, *, #2253, .F. ) ;
#4743=EDGE_CURVE ( 'NONE', #5437, #9732, #5208, .T. ) ;
#4766=VECTOR ( 'NONE', #4450, 1000.000000000000000 ) ;
#4771=ORIENTED_EDGE ( 'NONE', *, *, #8080, .F. ) ;
#4772=DIRECTION ( 'NONE',  ( 0.000000000000000000, 0.000000000000000000, -1.000000000000000000 ) ) ;
#4784=CARTESIAN_POINT ( 'NONE',  ( 53.33333333333330017, -20.00000000000000000, 225.1500000000000625 ) ) ;
#4791=EDGE_CURVE ( 'NONE', #4280, #9652, #5330, .T. ) ;
#4798=LINE ( 'NONE', #12554, #8979 ) ;
#4799=ORIENTED_EDGE ( 'NONE', *, *, #1343, .F. ) ;
#4801=VECTOR ( 'NONE', #11055, 1000.000000000000000 ) ;
#4808=AXIS2_PLACEMENT_3D ( 'NONE', #1374, #2765, #1513 ) ;
#4811=FACE_BOUND ( 'NONE', #14009, .T. ) ;
#4818=CARTESIAN_POINT ( 'NONE',  ( 132.4999999999999432, -56.99999999999997158, -180.0000000000000000 ) ) ;
#4827=EDGE_CURVE ( 'NONE', #5470, #8867, #1927, .T. ) ;
#4831=EDGE_CURVE ( 'NONE', #10300, #9742, #5138, .T. ) ;
#4834=AXIS2_PLACEMENT_3D ( 'NONE', #5134, #7576, #1768 ) ;
#4835=CYLINDRICAL_SURFACE ( 'NONE', #4625, 2.649999999999985700 ) ;
#4839=DIRECTION ( 'NONE',  ( -0.000000000000000000, -0.000000000000000000, 1.000000000000000000 ) ) ;
#4850=DIRECTION ( 'NONE',  ( -1.000000000000000000, 0.000000000000000000, 0.000000000000000000 ) ) ;
#4852=ADVANCED_FACE ( 'NONE', ( #11725 ), #6069, .F. ) ;
#4854=EDGE_LOOP ( 'NONE', ( #8838, #8501 ) ) ;
#4855=CARTESIAN_POINT ( 'NONE',  ( 299.9999999999999432, -75.00000000000008527, -186.2999999999999829 ) ) ;
#4858=VECTOR ( 'NONE', #8307, 1000.000000000000000 ) ;
#4866=ORIENTED_EDGE ( 'NONE', *, *, #9865, .F. ) ;
#4872=VECTOR ( 'NONE', #9268, 1000.000000000000000 ) ;
#4874=FACE_OUTER_BOUND ( 'NONE', #8626, .T. ) ;
#4880=FACE_BOUND ( 'NONE', #8930, .T. ) ;
#4881=ADVANCED_FACE ( 'NONE', ( #1855 ), #13028, .F. ) ;
#4889=ORIENTED_EDGE ( 'NONE', *, *, #10798, .F. ) ;
#4890=CARTESIAN_POINT ( 'NONE',  ( 134.9999999999999432, -36.99999999999997868, -169.9999999999999716 ) ) ;
#4892=CARTESIAN_POINT ( 'NONE',  ( 134.5000000000000000, -95.00000000000008527, -186.2999999999999829 ) ) ;
#4893=ORIENTED_EDGE ( 'NONE', *, *, #12085, .F. ) ;
#4895=DIRECTION ( 'NONE',  ( -0.000000000000000000, 1.000000000000000000, -0.000000000000000000 ) ) ;
#4901=CARTESIAN_POINT ( 'NONE',  ( 140.0000000000000000, -95.00000000000008527, -186.2999999999999829 ) ) ;
#4904=ORIENTED_EDGE ( 'NONE', *, *, #234, .T. ) ;
#4906=ADVANCED_FACE ( 'NONE', ( #11657 ), #5531, .F. ) ;
#4913=VECTOR ( 'NONE', #357, 1000.000000000000000 ) ;
#4914=CYLINDRICAL_SURFACE ( 'NONE', #12436, 2.649999999999985700 ) ;
#4920=EDGE_LOOP ( 'NONE', ( #51, #9218, #9560, #4048 ) ) ;
#4929=CARTESIAN_POINT ( 'NONE',  ( 140.0000000000000000, -95.00000000000008527, 186.2999999999999829 ) ) ;
#4930=CARTESIAN_POINT ( 'NONE',  ( 53.33333333333330017, -20.00000000000000000, 222.5000000000000853 ) ) ;
#4932=LINE ( 'NONE', #13763, #12898 ) ;
#4936=CYLINDRICAL_SURFACE ( 'NONE', #12256, 2.649999999999985700 ) ;
#4954=EDGE_CURVE ( 'NONE', #8236, #701, #8749, .T. ) ;
#4957=DIRECTION ( 'NONE',  ( -0.000000000000000000, -0.000000000000000000, 1.000000000000000000 ) ) ;
#4958=EDGE_LOOP ( 'NONE', ( #4247, #9694, #5845, #5829 ) ) ;
#4959=VERTEX_POINT ( 'NONE', #1995 ) ;
#4968=CARTESIAN_POINT ( 'NONE',  ( 53.33333333333330017, -20.00000000000000000, -225.1500000000000625 ) ) ;
#4970=LINE ( 'NONE', #580, #7208 ) ;
#4978=ORIENTED_EDGE ( 'NONE', *, *, #1252, .T. ) ;
#4983=ORIENTED_EDGE ( 'NONE', *, *, #1110, .F. ) ;
#4984=CARTESIAN_POINT ( 'NONE',  ( 305.4999999999999432, -95.00000000000008527, -186.2999999999999829 ) ) ;
#4989=CARTESIAN_POINT ( 'NONE',  ( 319.9999999999999432, -24.99999999999999289, 19.99999999999998934 ) ) ;
#4991=ORIENTED_EDGE ( 'NONE', *, *, #9026, .T. ) ;
#5003=EDGE_CURVE ( 'NONE', #5319, #13651, #6575, .T. ) ;
#5016=DIRECTION ( 'NONE',  ( 0.000000000000000000, 0.000000000000000000, -1.000000000000000000 ) ) ;
#5020=DIRECTION ( 'NONE',  ( 1.000000000000000000, 0.000000000000000000, 0.000000000000000000 ) ) ;
#5024=DIRECTION ( 'NONE',  ( 1.000000000000000000, 0.000000000000000000, 0.000000000000000000 ) ) ;
#5026=AXIS2_PLACEMENT_3D ( 'NONE', #10047, #70, #3381 ) ;
#5034=CARTESIAN_POINT ( 'NONE',  ( 134.9999999999999432, -36.99999999999997868, -180.0000000000000000 ) ) ;
#5037=EDGE_CURVE ( 'NONE', #7333, #13531, #13, .T. ) ;
#5038=VERTEX_POINT ( 'NONE', #11000 ) ;
#5045=VECTOR ( 'NONE', #1820, 1000.000000000000000 ) ;
#5046=CARTESIAN_POINT ( 'NONE',  ( 319.9999999999999432, -24.99999999999999289, -19.99999999999998934 ) ) ;
#5047=LINE ( 'NONE', #358, #3962 ) ;
#5054=DIRECTION ( 'NONE',  ( -0.000000000000000000, 1.000000000000000000, -0.000000000000000000 ) ) ;
#5057=ORIENTED_EDGE ( 'NONE', *, *, #5908, .T. ) ;
#5058=DIRECTION ( 'NONE',  ( -0.000000000000000000, 0.000000000000000000, 1.000000000000000000 ) ) ;
#5064=CARTESIAN_POINT ( 'NONE',  ( 302.5000000000000000, -56.99999999999997158, -180.0000000000000000 ) ) ;
#5065=EDGE_CURVE ( 'NONE', #2338, #770, #12087, .T. ) ;
#5069=DIRECTION ( 'NONE',  ( -0.000000000000000000, -0.000000000000000000, -1.000000000000000000 ) ) ;
#5071=ORIENTED_EDGE ( 'NONE', *, *, #872, .T. ) ;
#5077=DIRECTION ( 'NONE',  ( 1.000000000000000000, 0.000000000000000000, 0.000000000000000000 ) ) ;
#5078=DIRECTION ( 'NONE',  ( 0.000000000000000000, 0.000000000000000000, -1.000000000000000000 ) ) ;
#5079=ADVANCED_FACE ( 'NONE', ( #1397 ), #4835, .F. ) ;
#5084=DIRECTION ( 'NONE',  ( -0.000000000000000000, -0.000000000000000000, 1.000000000000000000 ) ) ;
#5091=EDGE_CURVE ( 'NONE', #3111, #11223, #11281, .T. ) ;
#5092=EDGE_CURVE ( 'NONE', #2372, #1020, #195, .T. ) ;
#5100=DIRECTION ( 'NONE',  ( -1.000000000000000000, 0.000000000000000000, 0.000000000000000000 ) ) ;
#5109=ORIENTED_EDGE ( 'NONE', *, *, #1687, .T. ) ;
#5111=EDGE_LOOP ( 'NONE', ( #10886, #4561 ) ) ;
#5112=CIRCLE ( 'NONE', #1849, 2.649999999999985700 ) ;
#5113=DIRECTION ( 'NONE',  ( -0.000000000000000000, 1.000000000000000000, -0.000000000000000000 ) ) ;
#5118=CYLINDRICAL_SURFACE ( 'NONE', #12664, 5.500000000000005329 ) ;
#5120=DIRECTION ( 'NONE',  ( 1.000000000000000000, 0.000000000000000000, 0.000000000000000000 ) ) ;
#5121=DIRECTION ( 'NONE',  ( -0.000000000000000000, -0.000000000000000000, 1.000000000000000000 ) ) ;
#5123=( NAMED_UNIT ( * ) PLANE_ANGLE_UNIT ( ) SI_UNIT ( $, .RADIAN. ) );
#5132=CARTESIAN_POINT ( 'NONE',  ( 229.9999999999999716, -85.00000000000007105, 190.0000000000000000 ) ) ;
#5134=CARTESIAN_POINT ( 'NONE',  ( -30.00000000000002842, -225.0000000000000000, 190.0000000000000000 ) ) ;
#5135=EDGE_LOOP ( 'NONE', ( #13233, #9452 ) ) ;
#5138=LINE ( 'NONE', #4038, #660 ) ;
#5145=DIRECTION ( 'NONE',  ( -0.000000000000000000, -0.000000000000000000, 1.000000000000000000 ) ) ;
#5146=CARTESIAN_POINT ( 'NONE',  ( 469.9999999999998863, -225.0000000000000000, -190.0000000000000000 ) ) ;
#5155=CARTESIAN_POINT ( 'NONE',  ( 140.0000000000000000, -75.00000000000008527, -186.2999999999999829 ) ) ;
#5164=EDGE_CURVE ( 'NONE', #3114, #9120, #1815, .T. ) ;
#5166=ORIENTED_EDGE ( 'NONE', *, *, #2777, .T. ) ;
#5168=ORIENTED_EDGE ( 'NONE', *, *, #1169, .T. ) ;
#5169=LINE ( 'NONE', #12913, #2225 ) ;
#5173=EDGE_CURVE ( 'NONE', #2036, #5508, #5906, .T. ) ;
#5175=CYLINDRICAL_SURFACE ( 'NONE', #13803, 2.500000000000002220 ) ;
#5185=EDGE_LOOP ( 'NONE', ( #9594, #347 ) ) ;
#5186=CARTESIAN_POINT ( 'NONE',  ( 219.9999999999999716, -25.00000000000000000, -225.1500000000000625 ) ) ;
#5188=ORIENTED_EDGE ( 'NONE', *, *, #1501, .F. ) ;
#5190=ORIENTED_EDGE ( 'NONE', *, *, #8080, .T. ) ;
#5192=EDGE_LOOP ( 'NONE', ( #268, #7880, #13626, #4542 ) ) ;
#5193=CARTESIAN_POINT ( 'NONE',  ( 299.9999999999999432, -95.00000000000008527, -169.9999999999999716 ) ) ;
#5208=LINE ( 'NONE', #9554, #183 ) ;
#5227=ORIENTED_EDGE ( 'NONE', *, *, #7894, .F. ) ;
#5229=CYLINDRICAL_SURFACE ( 'NONE', #2318, 2.649999999999985700 ) ;
#5235=ORIENTED_EDGE ( 'NONE', *, *, #9106, .F. ) ;
#5239=EDGE_CURVE ( 'NONE', #1677, #12041, #9027, .T. ) ;
#5243=EDGE_CURVE ( 'NONE', #12400, #13943, #10657, .T. ) ;
#5250=EDGE_LOOP ( 'NONE', ( #11925, #12792, #12559, #13482 ) ) ;
#5255=CIRCLE ( 'NONE', #9171, 2.649999999999985700 ) ;
#5257=CARTESIAN_POINT ( 'NONE',  ( 53.33333333333330017, -20.00000000000000000, 219.8500000000001080 ) ) ;
#5265=ORIENTED_EDGE ( 'NONE', *, *, #800, .T. ) ;
#5267=ORIENTED_EDGE ( 'NONE', *, *, #9608, .T. ) ;
#5275=DIRECTION ( 'NONE',  ( 1.000000000000000000, 0.000000000000000000, 0.000000000000000000 ) ) ;
#5281=EDGE_CURVE ( 'NONE', #12345, #11223, #11094, .T. ) ;
#5283=CARTESIAN_POINT ( 'NONE',  ( 201.0000000000000000, -85.00000000000007105, 190.0000000000000000 ) ) ;
#5300=ADVANCED_FACE ( 'NONE', ( #804 ), #2721, .F. ) ;
#5308=ORIENTED_EDGE ( 'NONE', *, *, #2479, .F. ) ;
#5314=DIRECTION ( 'NONE',  ( -0.000000000000000000, -0.000000000000000000, 1.000000000000000000 ) ) ;
#5316=VERTEX_POINT ( 'NONE', #14018 ) ;
#5319=VERTEX_POINT ( 'NONE', #581 ) ;
#5320=DIRECTION ( 'NONE',  ( -0.000000000000000000, 1.000000000000000000, -0.000000000000000000 ) ) ;
#5321=AXIS2_PLACEMENT_3D ( 'NONE', #3402, #1120, #5567 ) ;
#5322=VERTEX_POINT ( 'NONE', #8294 ) ;
#5324=CARTESIAN_POINT ( 'NONE',  ( 136.6666666666666288, -25.00000000000000000, -219.8500000000001080 ) ) ;
#5328=LINE ( 'NONE', #10910, #9680 ) ;
#5329=DIRECTION ( 'NONE',  ( 1.000000000000000000, 0.000000000000000000, 0.000000000000000000 ) ) ;
#5330=CIRCLE ( 'NONE', #13417, 2.649999999999985700 ) ;
#5334=AXIS2_PLACEMENT_3D ( 'NONE', #9576, #12022, #11949 ) ;
#5335=VERTEX_POINT ( 'NONE', #13951 ) ;
#5336=CARTESIAN_POINT ( 'NONE',  ( 386.6666666666666288, -20.00000000000000000, 219.8500000000001080 ) ) ;
#5338=DIRECTION ( 'NONE',  ( 0.000000000000000000, 0.000000000000000000, -1.000000000000000000 ) ) ;
#5341=FACE_OUTER_BOUND ( 'NONE', #1001, .T. ) ;
#5355=ORIENTED_EDGE ( 'NONE', *, *, #164, .T. ) ;
#5360=VECTOR ( 'NONE', #6855, 1000.000000000000000 ) ;
#5361=FACE_OUTER_BOUND ( 'NONE', #2024, .T. ) ;
#5364=APPLICATION_CONTEXT ( 'automotive_design' ) ;
#5365=VECTOR ( 'NONE', #8822, 1000.000000000000000 ) ;
#5373=ORIENTED_EDGE ( 'NONE', *, *, #3151, .F. ) ;
#5378=CARTESIAN_POINT ( 'NONE',  ( -30.00000000000002842, -25.00000000000000000, 250.0000000000000000 ) ) ;
#5386=VERTEX_POINT ( 'NONE', #8587 ) ;
#5387=DIRECTION ( 'NONE',  ( -0.000000000000000000, -0.000000000000000000, 1.000000000000000000 ) ) ;
#5389=DIRECTION ( 'NONE',  ( -0.000000000000000000, -0.000000000000000000, 1.000000000000000000 ) ) ;
#5396=CARTESIAN_POINT ( 'NONE',  ( 303.3333333333333144, -20.00000000000000000, 222.5000000000000853 ) ) ;
#5402=AXIS2_PLACEMENT_3D ( 'NONE', #9214, #5733, #10372 ) ;
#5404=DIRECTION ( 'NONE',  ( 0.000000000000000000, 1.000000000000000000, 0.000000000000000000 ) ) ;
#5411=ORIENTED_EDGE ( 'NONE', *, *, #12085, .T. ) ;
#5412=DIRECTION ( 'NONE',  ( -0.000000000000000000, 1.000000000000000000, -0.000000000000000000 ) ) ;
#5421=EDGE_CURVE ( 'NONE', #13943, #12400, #6877, .T. ) ;
#5422=EDGE_LOOP ( 'NONE', ( #7007, #40, #5645, #6400 ) ) ;
#5424=LINE ( 'NONE', #9846, #3510 ) ;
#5425=ORIENTED_EDGE ( 'NONE', *, *, #7150, .T. ) ;
#5430=ADVANCED_FACE ( 'NONE', ( #3162 ), #6626, .F. ) ;
#5432=DIRECTION ( 'NONE',  ( 0.000000000000000000, 0.000000000000000000, -1.000000000000000000 ) ) ;
#5435=CARTESIAN_POINT ( 'NONE',  ( 140.0000000000000000, -75.00000000000008527, -190.0000000000000000 ) ) ;
#5437=VERTEX_POINT ( 'NONE', #6560 ) ;
#5443=CARTESIAN_POINT ( 'NONE',  ( 134.9999999999999432, -36.99999999999997868, -169.9999999999999716 ) ) ;
#5448=CARTESIAN_POINT ( 'NONE',  ( 319.9999999999999432, -20.00000000000000000, -19.99999999999998934 ) ) ;
#5452=VECTOR ( 'NONE', #2330, 1000.000000000000000 ) ;
#5453=ORIENTED_EDGE ( 'NONE', *, *, #2224, .T. ) ;
#5455=EDGE_LOOP ( 'NONE', ( #1759, #5168, #3063 ) ) ;
#5470=VERTEX_POINT ( 'NONE', #5614 ) ;
#5477=DIRECTION ( 'NONE',  ( -0.000000000000000000, 1.000000000000000000, -0.000000000000000000 ) ) ;
#5481=DIRECTION ( 'NONE',  ( 0.000000000000000000, 0.000000000000000000, 1.000000000000000000 ) ) ;
#5482=VECTOR ( 'NONE', #13650, 1000.000000000000000 ) ;
#5484=EDGE_CURVE ( 'NONE', #9676, #5579, #5965, .T. ) ;
#5491=CARTESIAN_POINT ( 'NONE',  ( 142.6500000000000057, -95.00000000000008527, 169.9999999999999716 ) ) ;
#5502=DIRECTION ( 'NONE',  ( -0.000000000000000000, 1.000000000000000000, -0.000000000000000000 ) ) ;
#5504=VERTEX_POINT ( 'NONE', #9895 ) ;
#5508=VERTEX_POINT ( 'NONE', #4458 ) ;
#5518=DIRECTION ( 'NONE',  ( -0.000000000000000000, 1.000000000000000000, -0.000000000000000000 ) ) ;
#5520=DIRECTION ( 'NONE',  ( -1.000000000000000000, 0.000000000000000000, 0.000000000000000000 ) ) ;
#5524=ORIENTED_EDGE ( 'NONE', *, *, #11448, .F. ) ;
#5529=EDGE_CURVE ( 'NONE', #7333, #14219, #6769, .T. ) ;
#5530=FACE_OUTER_BOUND ( 'NONE', #3989, .T. ) ;
#5531=CONICAL_SURFACE ( 'NONE', #7634, 2.500000000000002220, 1.029744260000002631 ) ;
#5544=ORIENTED_EDGE ( 'NONE', *, *, #13322, .T. ) ;
#5548=CARTESIAN_POINT ( 'NONE',  ( 297.3499999999999659, -95.00000000000008527, -186.2999999999999829 ) ) ;
#5551=AXIS2_PLACEMENT_3D ( 'NONE', #29, #6518, #2227 ) ;
#5561=CARTESIAN_POINT ( 'NONE',  ( -30.00000000000002842, -25.00000000000000000, -169.9999999999999716 ) ) ;
#5567=DIRECTION ( 'NONE',  ( -1.000000000000000000, 0.000000000000000000, 0.000000000000000000 ) ) ;
#5572=VERTEX_POINT ( 'NONE', #9229 ) ;
#5574=CARTESIAN_POINT ( 'NONE',  ( 470.0000000000000000, -20.00000000000000000, 250.0000000000000000 ) ) ;
#5577=EDGE_CURVE ( 'NONE', #9015, #11802, #9450, .T. ) ;
#5579=VERTEX_POINT ( 'NONE', #10100 ) ;
#5582=DIRECTION ( 'NONE',  ( 1.000000000000000000, 0.000000000000000000, 0.000000000000000000 ) ) ;
#5584=AXIS2_PLACEMENT_3D ( 'NONE', #11491, #2719, #6052 ) ;
#5593=EDGE_CURVE ( 'NONE', #11304, #11403, #12489, .T. ) ;
#5602=ORIENTED_EDGE ( 'NONE', *, *, #614, .F. ) ;
#5605=VECTOR ( 'NONE', #7242, 1000.000000000000000 ) ;
#5612=DIRECTION ( 'NONE',  ( 1.000000000000000000, 0.000000000000000000, 0.000000000000000000 ) ) ;
#5613=CARTESIAN_POINT ( 'NONE',  ( 386.6666666666666288, -25.00000000000000000, -222.5000000000000853 ) ) ;
#5614=CARTESIAN_POINT ( 'NONE',  ( 201.0000000000000000, -85.00000000000007105, 180.0000000000000000 ) ) ;
#5623=CIRCLE ( 'NONE', #8627, 2.649999999999985700 ) ;
#5626=EDGE_CURVE ( 'NONE', #13531, #3034, #3444, .T. ) ;
#5627=CARTESIAN_POINT ( 'NONE',  ( 219.9999999999999716, -20.00000000000000000, -225.1500000000000625 ) ) ;
#5631=DIRECTION ( 'NONE',  ( 1.000000000000000000, 0.000000000000000000, 0.000000000000000000 ) ) ;
#5633=ADVANCED_FACE ( 'NONE', ( #13428, #1456, #342, #8128, #4811, #10173, #12565, #12354, #7845, #12417, #2632, #7049, #11476 ), #10041, .T. ) ;
#5634=ORIENTED_EDGE ( 'NONE', *, *, #1080, .F. ) ;
#5645=ORIENTED_EDGE ( 'NONE', *, *, #7023, .T. ) ;
#5648=EDGE_LOOP ( 'NONE', ( #8369, #11246, #6545, #654 ) ) ;
#5650=CARTESIAN_POINT ( 'NONE',  ( 236.4999999999999432, -85.00000000000007105, 178.4978484569338946 ) ) ;
#5651=DIRECTION ( 'NONE',  ( -0.000000000000000000, -0.000000000000000000, 1.000000000000000000 ) ) ;
#5653=FACE_BOUND ( 'NONE', #1931, .T. ) ;
#5655=CARTESIAN_POINT ( 'NONE',  ( 299.9999999999999432, -75.00000000000008527, -169.9999999999999716 ) ) ;
#5657=LINE ( 'NONE', #111, #9246 ) ;
#5662=LINE ( 'NONE', #12478, #4467 ) ;
#5668=DIRECTION ( 'NONE',  ( -0.000000000000000000, 1.000000000000000000, -0.000000000000000000 ) ) ;
#5670=ADVANCED_FACE ( 'NONE', ( #6834 ), #7977, .F. ) ;
#5673=ADVANCED_FACE ( 'NONE', ( #6034 ), #11620, .F. ) ;
#5676=ORIENTED_EDGE ( 'NONE', *, *, #7087, .T. ) ;
#5684=AXIS2_PLACEMENT_3D ( 'NONE', #3198, #10881, #2092 ) ;
#5688=DIRECTION ( 'NONE',  ( 1.000000000000000000, 0.000000000000000000, 0.000000000000000000 ) ) ;
#5694=EDGE_CURVE ( 'NONE', #10615, #1243, #9375, .T. ) ;
#5696=DIRECTION ( 'NONE',  ( 0.000000000000000000, 0.000000000000000000, 1.000000000000000000 ) ) ;
#5698=LINE ( 'NONE', #1192, #7354 ) ;
#5699=ORIENTED_EDGE ( 'NONE', *, *, #5774, .F. ) ;
#5713=ORIENTED_EDGE ( 'NONE', *, *, #4069, .F. ) ;
#5715=DIRECTION ( 'NONE',  ( 0.000000000000000000, 0.000000000000000000, -1.000000000000000000 ) ) ;
#5718=FACE_OUTER_BOUND ( 'NONE', #4679, .T. ) ;
#5719=LINE ( 'NONE', #2455, #6730 ) ;
#5721=CARTESIAN_POINT ( 'NONE',  ( 119.9999999999999147, -225.0010000000000048, -169.9999999999999716 ) ) ;
#5726=AXIS2_PLACEMENT_3D ( 'NONE', #3501, #197, #5950 ) ;
#5729=ORIENTED_EDGE ( 'NONE', *, *, #7357, .T. ) ;
#5730=DIRECTION ( 'NONE',  ( -1.000000000000000000, 0.000000000000000000, 0.000000000000000000 ) ) ;
#5732=ORIENTED_EDGE ( 'NONE', *, *, #9957, .T. ) ;
#5733=DIRECTION ( 'NONE',  ( 0.000000000000000000, 1.000000000000000000, 0.000000000000000000 ) ) ;
#5734=CONICAL_SURFACE ( 'NONE', #6895, 2.500000000000002220, 1.029744260000002631 ) ;
#5735=ORIENTED_EDGE ( 'NONE', *, *, #1501, .T. ) ;
#5736=DIRECTION ( 'NONE',  ( 0.000000000000000000, 0.000000000000000000, -1.000000000000000000 ) ) ;
#5747=EDGE_LOOP ( 'NONE', ( #7622, #4444, #13530, #9438 ) ) ;
#5760=CIRCLE ( 'NONE', #3003, 2.649999999999985700 ) ;
#5768=CARTESIAN_POINT ( 'NONE',  ( -30.00000000000002842, -20.00000000000000000, 250.0000000000000000 ) ) ;
#5769=AXIS2_PLACEMENT_3D ( 'NONE', #12239, #10063, #1266 ) ;
#5774=EDGE_CURVE ( 'NONE', #7639, #13552, #2023, .T. ) ;
#5775=ADVANCED_FACE ( 'NONE', ( #1740, #12923 ), #7332, .F. ) ;
#5783=ORIENTED_EDGE ( 'NONE', *, *, #9393, .T. ) ;
#5785=ORIENTED_EDGE ( 'NONE', *, *, #7456, .T. ) ;
#5786=DIRECTION ( 'NONE',  ( -0.000000000000000000, -0.000000000000000000, 1.000000000000000000 ) ) ;
#5787=ORIENTED_EDGE ( 'NONE', *, *, #947, .T. ) ;
#5789=CARTESIAN_POINT ( 'NONE',  ( 53.33333333333330017, -25.00000000000000000, -219.8500000000001080 ) ) ;
#5794=CARTESIAN_POINT ( 'NONE',  ( 132.4999999999999432, -36.99999999999997868, -180.0000000000000000 ) ) ;
#5798=CIRCLE ( 'NONE', #8821, 2.649999999999985700 ) ;
#5801=EDGE_LOOP ( 'NONE', ( #1226, #3435, #11245, #4713 ) ) ;
#5803=EDGE_CURVE ( 'NONE', #9645, #1558, #13152, .T. ) ;
#5809=CARTESIAN_POINT ( 'NONE',  ( 53.33333333333330017, -20.00000000000000000, -222.5000000000000853 ) ) ;
#5811=MECHANICAL_DESIGN_GEOMETRIC_PRESENTATION_REPRESENTATION('',(#12530),#14150);
#5817=CIRCLE ( 'NONE', #7663, 2.500000000000002220 ) ;
#5819=DIRECTION ( 'NONE',  ( 1.000000000000000000, 0.000000000000000000, 0.000000000000000000 ) ) ;
#5821=EDGE_LOOP ( 'NONE', ( #6114, #3410, #8132, #14019, #8765, #9726, #6184, #12654, #4076, #7270, #9982, #1944 ) ) ;
#5824=DIRECTION ( 'NONE',  ( 0.000000000000000000, 0.000000000000000000, 1.000000000000000000 ) ) ;
#5829=ORIENTED_EDGE ( 'NONE', *, *, #2230, .T. ) ;
#5832=DIRECTION ( 'NONE',  ( -0.000000000000000000, -0.000000000000000000, 1.000000000000000000 ) ) ;
#5835=DIRECTION ( 'NONE',  ( -0.000000000000000000, -0.000000000000000000, 1.000000000000000000 ) ) ;
#5838=CARTESIAN_POINT ( 'NONE',  ( 136.6666666666666288, -20.00000000000000000, 222.5000000000000853 ) ) ;
#5842=LINE ( 'NONE', #11571, #7878 ) ;
#5845=ORIENTED_EDGE ( 'NONE', *, *, #7366, .T. ) ;
#5847=DIRECTION ( 'NONE',  ( 0.000000000000000000, 0.000000000000000000, 1.000000000000000000 ) ) ;
#5853=CIRCLE ( 'NONE', #13964, 2.649999999999985700 ) ;
#5856=AXIS2_PLACEMENT_3D ( 'NONE', #13608, #10350, #3971 ) ;
#5857=ORIENTED_EDGE ( 'NONE', *, *, #3151, .T. ) ;
#5868=LINE ( 'NONE', #9204, #11061 ) ;
#5871=VERTEX_POINT ( 'NONE', #1000 ) ;
#5872=VERTEX_POINT ( 'NONE', #5448 ) ;
#5882=EDGE_CURVE ( 'NONE', #5322, #2121, #14265, .T. ) ;
#5883=CARTESIAN_POINT ( 'NONE',  ( 219.9999999999999716, -20.00000000000000000, 222.5000000000000853 ) ) ;
#5892=ORIENTED_EDGE ( 'NONE', *, *, #3914, .F. ) ;
#5895=ORIENTED_EDGE ( 'NONE', *, *, #2122, .T. ) ;
#5899=ORIENTED_EDGE ( 'NONE', *, *, #6398, .T. ) ;
#5900=DIRECTION ( 'NONE',  ( 0.000000000000000000, 1.000000000000000000, 0.000000000000000000 ) ) ;
#5902=DIRECTION ( 'NONE',  ( 1.000000000000000000, 0.000000000000000000, 0.000000000000000000 ) ) ;
#5904=LINE ( 'NONE', #10326, #4913 ) ;
#5905=CYLINDRICAL_SURFACE ( 'NONE', #11609, 5.500000000000005329 ) ;
#5906=LINE ( 'NONE', #12509, #13655 ) ;
#5908=EDGE_CURVE ( 'NONE', #1839, #3111, #6170, .T. ) ;
#5911=VECTOR ( 'NONE', #2617, 1000.000000000000000 ) ;
#5918=DIRECTION ( 'NONE',  ( -0.000000000000000000, -1.000000000000000000, -0.000000000000000000 ) ) ;
#5927=VERTEX_POINT ( 'NONE', #782 ) ;
#5933=DIRECTION ( 'NONE',  ( 1.000000000000000000, 0.000000000000000000, 0.000000000000000000 ) ) ;
#5937=VECTOR ( 'NONE', #5518, 1000.000000000000000 ) ;
#5939=CIRCLE ( 'NONE', #4093, 5.500000000000005329 ) ;
#5944=EDGE_LOOP ( 'NONE', ( #13398, #9961, #9917, #9595 ) ) ;
#5946=EDGE_CURVE ( 'NONE', #4174, #13795, #13108, .T. ) ;
#5950=DIRECTION ( 'NONE',  ( -1.000000000000000000, 0.000000000000000000, 0.000000000000000000 ) ) ;
#5951=EDGE_LOOP ( 'NONE', ( #11327, #3252, #13727 ) ) ;
#5955=EDGE_LOOP ( 'NONE', ( #2204, #13752 ) ) ;
#5965=CIRCLE ( 'NONE', #1780, 2.500000000000002220 ) ;
#5973=AXIS2_PLACEMENT_3D ( 'NONE', #7257, #1733, #5100 ) ;
#5977=CARTESIAN_POINT ( 'NONE',  ( 119.9999999999999147, -24.99999999999999289, -19.99999999999998934 ) ) ;
#5987=( LENGTH_UNIT ( ) NAMED_UNIT ( * ) SI_UNIT ( .MILLI., .METRE. ) );
#5988=CARTESIAN_POINT ( 'NONE',  ( 236.4999999999999432, -85.00000000000007105, 190.0000000000000000 ) ) ;
#5990=DIRECTION ( 'NONE',  ( -0.000000000000000000, -1.000000000000000000, -0.000000000000000000 ) ) ;
#5993=DIRECTION ( 'NONE',  ( -1.000000000000000000, 0.000000000000000000, 0.000000000000000000 ) ) ;
#5998=ORIENTED_EDGE ( 'NONE', *, *, #7276, .T. ) ;
#6003=ORIENTED_EDGE ( 'NONE', *, *, #10557, .T. ) ;
#6005=CARTESIAN_POINT ( 'NONE',  ( 137.3500000000000227, -75.00000000000008527, -186.2999999999999829 ) ) ;
#6008=DIRECTION ( 'NONE',  ( 0.000000000000000000, 0.000000000000000000, -1.000000000000000000 ) ) ;
#6014=ORIENTED_EDGE ( 'NONE', *, *, #12358, .T. ) ;
#6020=ORIENTED_EDGE ( 'NONE', *, *, #13161, .T. ) ;
#6022=ORIENTED_EDGE ( 'NONE', *, *, #2424, .T. ) ;
#6023=CIRCLE ( 'NONE', #7178, 2.500000000000002220 ) ;
#6024=DIRECTION ( 'NONE',  ( -1.000000000000000000, 0.000000000000000000, 0.000000000000000000 ) ) ;
#6025=DIRECTION ( 'NONE',  ( 0.000000000000000000, 0.000000000000000000, -1.000000000000000000 ) ) ;
#6028=FACE_OUTER_BOUND ( 'NONE', #6349, .T. ) ;
#6031=CARTESIAN_POINT ( 'NONE',  ( 233.9999999999999432, -85.00000000000007105, 190.0000000000000000 ) ) ;
#6034=FACE_OUTER_BOUND ( 'NONE', #5747, .T. ) ;
#6039=CIRCLE ( 'NONE', #7187, 10.00000000000000888 ) ;
#6042=VECTOR ( 'NONE', #9129, 1000.000000000000000 ) ;
#6044=VERTEX_POINT ( 'NONE', #4989 ) ;
#6050=CARTESIAN_POINT ( 'NONE',  ( 137.3500000000000227, -75.00000000000008527, -190.0000000000000000 ) ) ;
#6052=DIRECTION ( 'NONE',  ( 1.000000000000000000, 0.000000000000000000, 0.000000000000000000 ) ) ;
#6069=CYLINDRICAL_SURFACE ( 'NONE', #11130, 2.649999999999985700 ) ;
#6078=ORIENTED_EDGE ( 'NONE', *, *, #2777, .F. ) ;
#6092=ORIENTED_EDGE ( 'NONE', *, *, #2241, .T. ) ;
#6097=ORIENTED_EDGE ( 'NONE', *, *, #9936, .F. ) ;
#6100=DIRECTION ( 'NONE',  ( -0.000000000000000000, -0.000000000000000000, 1.000000000000000000 ) ) ;
#6108=ADVANCED_FACE ( 'NONE', ( #11510 ), #4508, .F. ) ;
#6110=ORIENTED_EDGE ( 'NONE', *, *, #5694, .T. ) ;
#6113=CARTESIAN_POINT ( 'NONE',  ( 386.6666666666666288, -25.00000000000000000, 225.1500000000000625 ) ) ;
#6114=ORIENTED_EDGE ( 'NONE', *, *, #6715, .F. ) ;
#6117=EDGE_CURVE ( 'NONE', #840, #13282, #6139, .T. ) ;
#6120=CARTESIAN_POINT ( 'NONE',  ( -30.00000000000002842, -225.0000000000000000, -190.0000000000000000 ) ) ;
#6122=CARTESIAN_POINT ( 'NONE',  ( 302.5000000000000000, -56.99999999999997158, -169.9999999999999716 ) ) ;
#6127=EDGE_LOOP ( 'NONE', ( #12285, #3154, #4677, #9672 ) ) ;
#6129=EDGE_LOOP ( 'NONE', ( #12707, #9544, #2444, #4866 ) ) ;
#6130=CARTESIAN_POINT ( 'NONE',  ( 134.9999999999999432, -56.99999999999997158, -180.0000000000000000 ) ) ;
#6139=LINE ( 'NONE', #1707, #4321 ) ;
#6143=ADVANCED_FACE ( 'NONE', ( #9872 ), #7564, .F. ) ;
#6144=EDGE_CURVE ( 'NONE', #9739, #5872, #108, .T. ) ;
#6146=LINE ( 'NONE', #3684, #4872 ) ;
#6148=EDGE_LOOP ( 'NONE', ( #1595, #4983 ) ) ;
#6150=AXIS2_PLACEMENT_3D ( 'NONE', #8266, #11682, #405 ) ;
#6160=AXIS2_PLACEMENT_3D ( 'NONE', #180, #4637, #2174 ) ;
#6168=CARTESIAN_POINT ( 'NONE',  ( 137.3500000000000227, -75.00000000000008527, 190.0000000000000000 ) ) ;
#6170=CIRCLE ( 'NONE', #12420, 2.649999999999985700 ) ;
#6171=CARTESIAN_POINT ( 'NONE',  ( 140.0000000000000000, -75.00000000000008527, 190.0000000000000000 ) ) ;
#6174=AXIS2_PLACEMENT_3D ( 'NONE', #3260, #7662, #12097 ) ;
#6176=DIRECTION ( 'NONE',  ( 0.000000000000000000, 0.000000000000000000, -1.000000000000000000 ) ) ;
#6184=ORIENTED_EDGE ( 'NONE', *, *, #4592, .T. ) ;
#6185=DIRECTION ( 'NONE',  ( 0.000000000000000000, 0.000000000000000000, 1.000000000000000000 ) ) ;
#6187=CARTESIAN_POINT ( 'NONE',  ( 299.9999999999999432, -95.00000000000008527, -190.0000000000000000 ) ) ;
#6192=FACE_BOUND ( 'NONE', #7484, .T. ) ;
#6201=ORIENTED_EDGE ( 'NONE', *, *, #11650, .F. ) ;
#6206=CARTESIAN_POINT ( 'NONE',  ( 305.0000000000000000, -36.99999999999997868, -169.9999999999999716 ) ) ;
#6207=FACE_BOUND ( 'NONE', #11539, .T. ) ;
#6209=CIRCLE ( 'NONE', #4598, 2.649999999999985700 ) ;
#6214=EDGE_CURVE ( 'NONE', #5872, #8099, #4366, .T. ) ;
#6219=CARTESIAN_POINT ( 'NONE',  ( 53.33333333333330017, -20.00000000000000000, -222.5000000000000853 ) ) ;
#6222=EDGE_CURVE ( 'NONE', #8495, #7265, #10819, .T. ) ;
#6223=ADVANCED_FACE ( 'NONE', ( #2180 ), #1068, .F. ) ;
#6227=DIRECTION ( 'NONE',  ( -0.000000000000000000, -0.000000000000000000, -1.000000000000000000 ) ) ;
#6228=DIRECTION ( 'NONE',  ( 0.000000000000000000, 1.000000000000000000, 0.000000000000000000 ) ) ;
#6231=ADVANCED_FACE ( 'NONE', ( #9947 ), #5175, .F. ) ;
#6238=VERTEX_POINT ( 'NONE', #47 ) ;
#6247=FACE_OUTER_BOUND ( 'NONE', #12982, .T. ) ;
#6248=EDGE_CURVE ( 'NONE', #1243, #9474, #8991, .T. ) ;
#6251=ORIENTED_EDGE ( 'NONE', *, *, #13379, .T. ) ;
#6252=AXIS2_PLACEMENT_3D ( 'NONE', #7859, #6789, #12437 ) ;
#6253=EDGE_LOOP ( 'NONE', ( #11118, #12440, #7626, #4032 ) ) ;
#6260=CARTESIAN_POINT ( 'NONE',  ( 233.9999999999999432, -85.00000000000007105, 190.0000000000000000 ) ) ;
#6261=DIRECTION ( 'NONE',  ( -0.000000000000000000, 1.000000000000000000, -0.000000000000000000 ) ) ;
#6263=CARTESIAN_POINT ( 'NONE',  ( 297.3499999999999659, -95.00000000000008527, 169.9999999999999716 ) ) ;
#6271=CARTESIAN_POINT ( 'NONE',  ( 219.9999999999999716, -20.00000000000000000, 222.5000000000000853 ) ) ;
#6275=FACE_BOUND ( 'NONE', #4251, .T. ) ;
#6278=DIRECTION ( 'NONE',  ( 0.000000000000000000, 1.000000000000000000, 0.000000000000000000 ) ) ;
#6281=CARTESIAN_POINT ( 'NONE',  ( 303.3333333333333144, -25.00000000000000000, 219.8500000000001080 ) ) ;
#6285=PLANE ( 'NONE',  #4197 ) ;
#6287=ORIENTED_EDGE ( 'NONE', *, *, #11567, .F. ) ;
#6288=CARTESIAN_POINT ( 'NONE',  ( 470.0000000000000000, -20.00000000000000000, -250.0000000000000000 ) ) ;
#6294=CYLINDRICAL_SURFACE ( 'NONE', #9179, 5.500000000000005329 ) ;
#6296=CARTESIAN_POINT ( 'NONE',  ( 303.3333333333333144, -20.00000000000000000, -219.8500000000001080 ) ) ;
#6301=ORIENTED_EDGE ( 'NONE', *, *, #11515, .F. ) ;
#6305=EDGE_LOOP ( 'NONE', ( #11992, #4067, #5998, #12317 ) ) ;
#6316=AXIS2_PLACEMENT_3D ( 'NONE', #6206, #2947, #11719 ) ;
#6318=DIRECTION ( 'NONE',  ( -0.000000000000000000, -0.000000000000000000, -1.000000000000000000 ) ) ;
#6325=CARTESIAN_POINT ( 'NONE',  ( 203.5000000000000000, -85.00000000000007105, 190.0000000000000000 ) ) ;
#6334=ORIENTED_EDGE ( 'NONE', *, *, #9790, .F. ) ;
#6336=EDGE_CURVE ( 'NONE', #12884, #12902, #9187, .T. ) ;
#6338=VERTEX_POINT ( 'NONE', #391 ) ;
#6339=ORIENTED_EDGE ( 'NONE', *, *, #8451, .T. ) ;
#6342=DIRECTION ( 'NONE',  ( -0.000000000000000000, -0.000000000000000000, 1.000000000000000000 ) ) ;
#6348=DIRECTION ( 'NONE',  ( -0.000000000000000000, -0.000000000000000000, -1.000000000000000000 ) ) ;
#6349=EDGE_LOOP ( 'NONE', ( #2926, #7079, #36, #13544 ) ) ;
#6354=FACE_BOUND ( 'NONE', #8517, .T. ) ;
#6356=LINE ( 'NONE', #12815, #4207 ) ;
#6360=LINE ( 'NONE', #2811, #3484 ) ;
#6370=DIRECTION ( 'NONE',  ( 1.000000000000000000, 0.000000000000000000, 0.000000000000000000 ) ) ;
#6374=VECTOR ( 'NONE', #8040, 1000.000000000000000 ) ;
#6380=PLANE ( 'NONE',  #9614 ) ;
#6382=DIRECTION ( 'NONE',  ( 1.000000000000000000, 0.000000000000000000, 0.000000000000000000 ) ) ;
#6383=DIRECTION ( 'NONE',  ( -0.000000000000000000, 1.000000000000000000, -0.000000000000000000 ) ) ;
#6387=LINE ( 'NONE', #10888, #8711 ) ;
#6388=CARTESIAN_POINT ( 'NONE',  ( 219.9999999999999716, -25.00000000000000000, -222.5000000000000853 ) ) ;
#6389=VERTEX_POINT ( 'NONE', #10437 ) ;
#6398=EDGE_CURVE ( 'NONE', #3114, #5927, #5868, .T. ) ;
#6400=ORIENTED_EDGE ( 'NONE', *, *, #6398, .F. ) ;
#6402=VERTEX_POINT ( 'NONE', #13539 ) ;
#6403=VERTEX_POINT ( 'NONE', #4784 ) ;
#6404=DIRECTION ( 'NONE',  ( 0.000000000000000000, 1.000000000000000000, 0.000000000000000000 ) ) ;
#6406=DIRECTION ( 'NONE',  ( 1.000000000000000000, 0.000000000000000000, 0.000000000000000000 ) ) ;
#6410=EDGE_CURVE ( 'NONE', #6238, #1677, #4932, .T. ) ;
#6415=CARTESIAN_POINT ( 'NONE',  ( 134.9999999999999432, -56.99999999999997158, -169.9999999999999716 ) ) ;
#6423=CARTESIAN_POINT ( 'NONE',  ( -30.00000000000002842, -25.00000000000000000, -250.0000000000000000 ) ) ;
#6425=CARTESIAN_POINT ( 'NONE',  ( 297.3499999999999659, -95.00000000000008527, 190.0000000000000000 ) ) ;
#6427=ORIENTED_EDGE ( 'NONE', *, *, #12971, .T. ) ;
#6428=CIRCLE ( 'NONE', #3194, 2.500000000000002220 ) ;
#6429=ADVANCED_FACE ( 'NONE', ( #11273 ), #4534, .F. ) ;
#6435=ORIENTED_EDGE ( 'NONE', *, *, #5164, .F. ) ;
#6441=CARTESIAN_POINT ( 'NONE',  ( 201.0000000000000000, -85.00000000000007105, 180.0000000000000000 ) ) ;
#6445=CARTESIAN_POINT ( 'NONE',  ( 305.4999999999999432, -95.00000000000008527, -190.0000000000000000 ) ) ;
#6449=CIRCLE ( 'NONE', #14087, 5.500000000000005329 ) ;
#6451=CARTESIAN_POINT ( 'NONE',  ( -30.00000000000002842, -225.0000000000000000, 169.9999999999999716 ) ) ;
#6454=LINE ( 'NONE', #9581, #2365 ) ;
#6455=LINE ( 'NONE', #9798, #7416 ) ;
#6458=EDGE_LOOP ( 'NONE', ( #1989, #10921, #12341, #12906 ) ) ;
#6462=LINE ( 'NONE', #7404, #4584 ) ;
#6478=AXIS2_PLACEMENT_3D ( 'NONE', #3713, #2411, #2697 ) ;
#6479=CYLINDRICAL_SURFACE ( 'NONE', #10322, 2.649999999999985700 ) ;
#6482=EDGE_CURVE ( 'NONE', #7600, #5508, #4468, .T. ) ;
#6485=CARTESIAN_POINT ( 'NONE',  ( 305.0000000000000000, -36.99999999999997868, -180.0000000000000000 ) ) ;
#6507=AXIS2_PLACEMENT_3D ( 'NONE', #7729, #5824, #3795 ) ;
#6514=EDGE_LOOP ( 'NONE', ( #8787, #10386, #7314, #7127 ) ) ;
#6517=VECTOR ( 'NONE', #229, 1000.000000000000000 ) ;
#6518=DIRECTION ( 'NONE',  ( 0.000000000000000000, 0.000000000000000000, -1.000000000000000000 ) ) ;
#6523=AXIS2_PLACEMENT_3D ( 'NONE', #3728, #1539, #288 ) ;
#6524=ORIENTED_EDGE ( 'NONE', *, *, #2672, .T. ) ;
#6525=CARTESIAN_POINT ( 'NONE',  ( 0.000000000000000000, -225.0000000000000000, 0.000000000000000000 ) ) ;
#6526=CYLINDRICAL_SURFACE ( 'NONE', #6719, 5.500000000000005329 ) ;
#6527=ORIENTED_EDGE ( 'NONE', *, *, #11731, .T. ) ;
#6528=ORIENTED_EDGE ( 'NONE', *, *, #10557, .F. ) ;
#6534=DIRECTION ( 'NONE',  ( 0.000000000000000000, -0.000000000000000000, 1.000000000000000000 ) ) ;
#6536=CARTESIAN_POINT ( 'NONE',  ( 299.9999999999999432, -75.00000000000008527, -190.0000000000000000 ) ) ;
#6542=ORIENTED_EDGE ( 'NONE', *, *, #7204, .T. ) ;
#6544=CYLINDRICAL_SURFACE ( 'NONE', #801, 2.649999999999985700 ) ;
#6545=ORIENTED_EDGE ( 'NONE', *, *, #5577, .F. ) ;
#6547=ORIENTED_EDGE ( 'NONE', *, *, #12747, .T. ) ;
#6550=CARTESIAN_POINT ( 'NONE',  ( 137.3500000000000227, -75.00000000000008527, 169.9999999999999716 ) ) ;
#6553=DIRECTION ( 'NONE',  ( 1.000000000000000000, 0.000000000000000000, 0.000000000000000000 ) ) ;
#6559=DIRECTION ( 'NONE',  ( 0.000000000000000000, 0.000000000000000000, -1.000000000000000000 ) ) ;
#6560=CARTESIAN_POINT ( 'NONE',  ( 134.5000000000000000, -75.00000000000008527, 186.2999999999999829 ) ) ;
#6569=DIRECTION ( 'NONE',  ( 1.000000000000000000, 0.000000000000000000, 0.000000000000000000 ) ) ;
#6572=APPLICATION_CONTEXT ( 'automotive_design' ) ;
#6574=CARTESIAN_POINT ( 'NONE',  ( 53.33333333333330017, -20.00000000000000000, 222.5000000000000853 ) ) ;
#6575=LINE ( 'NONE', #4478, #10887 ) ;
#6583=ORIENTED_EDGE ( 'NONE', *, *, #11718, .T. ) ;
#6586=ADVANCED_FACE ( 'NONE', ( #11632 ), #5118, .F. ) ;
#6592=ORIENTED_EDGE ( 'NONE', *, *, #11811, .F. ) ;
#6596=DIRECTION ( 'NONE',  ( 1.000000000000000000, 0.000000000000000000, -0.000000000000000000 ) ) ;
#6603=CARTESIAN_POINT ( 'NONE',  ( 145.5000000000000284, -95.00000000000008527, 190.0000000000000000 ) ) ;
#6612=EDGE_LOOP ( 'NONE', ( #1194, #1508, #11295, #6963 ) ) ;
#6614=EDGE_CURVE ( 'NONE', #14219, #3774, #10544, .T. ) ;
#6615=EDGE_LOOP ( 'NONE', ( #4771, #6998, #8572, #9527 ) ) ;
#6619=CARTESIAN_POINT ( 'NONE',  ( 140.0000000000000000, -95.00000000000008527, -190.0000000000000000 ) ) ;
#6623=FILL_AREA_STYLE ('',( #7975 ) ) ;
#6625=CARTESIAN_POINT ( 'NONE',  ( 53.33333333333330017, -25.00000000000000000, -225.1500000000000625 ) ) ;
#6626=CYLINDRICAL_SURFACE ( 'NONE', #12443, 2.649999999999985700 ) ;
#6627=ORIENTED_EDGE ( 'NONE', *, *, #2479, .T. ) ;
#6631=EDGE_LOOP ( 'NONE', ( #445, #4742 ) ) ;
#6633=FACE_OUTER_BOUND ( 'NONE', #10319, .T. ) ;
#6642=AXIS2_PLACEMENT_3D ( 'NONE', #9634, #13977, #2892 ) ;
#6652=ORIENTED_EDGE ( 'NONE', *, *, #9512, .F. ) ;
#6654=AXIS2_PLACEMENT_3D ( 'NONE', #7492, #8502, #2785 ) ;
#6658=FACE_BOUND ( 'NONE', #13900, .T. ) ;
#6662=CIRCLE ( 'NONE', #12450, 2.649999999999985700 ) ;
#6665=VERTEX_POINT ( 'NONE', #8208 ) ;
#6670=ORIENTED_EDGE ( 'NONE', *, *, #1080, .T. ) ;
#6671=DIRECTION ( 'NONE',  ( 0.000000000000000000, 0.000000000000000000, -1.000000000000000000 ) ) ;
#6672=VECTOR ( 'NONE', #6861, 1000.000000000000000 ) ;
#6677=CARTESIAN_POINT ( 'NONE',  ( 302.6499999999999204, -95.00000000000008527, 186.2999999999999829 ) ) ;
#6679=CARTESIAN_POINT ( 'NONE',  ( 319.9999999999999432, -225.0010000000000048, -19.99999999999998934 ) ) ;
#6684=EDGE_LOOP ( 'NONE', ( #1287, #1224 ) ) ;
#6688=EDGE_CURVE ( 'NONE', #13943, #7291, #12793, .T. ) ;
#6689=AXIS2_PLACEMENT_3D ( 'NONE', #1756, #6348, #11860 ) ;
#6690=ORIENTED_EDGE ( 'NONE', *, *, #3498, .F. ) ;
#6701=DIRECTION ( 'NONE',  ( -0.000000000000000000, -0.000000000000000000, 1.000000000000000000 ) ) ;
#6706=ORIENTED_EDGE ( 'NONE', *, *, #12747, .F. ) ;
#6707=CARTESIAN_POINT ( 'NONE',  ( 299.9999999999999432, -75.00000000000008527, -169.9999999999999716 ) ) ;
#6711=LINE ( 'NONE', #9837, #7891 ) ;
#6712=DIRECTION ( 'NONE',  ( -0.000000000000000000, -0.000000000000000000, -1.000000000000000000 ) ) ;
#6715=EDGE_CURVE ( 'NONE', #9739, #2036, #11485, .T. ) ;
#6716=VERTEX_POINT ( 'NONE', #13075 ) ;
#6719=AXIS2_PLACEMENT_3D ( 'NONE', #5435, #11023, #9859 ) ;
#6721=LINE ( 'NONE', #22, #3652 ) ;
#6730=VECTOR ( 'NONE', #10150, 1000.000000000000000 ) ;
#6731=EDGE_LOOP ( 'NONE', ( #6592, #10353 ) ) ;
#6736=EDGE_CURVE ( 'NONE', #10043, #7698, #6854, .T. ) ;
#6737=CONICAL_SURFACE ( 'NONE', #453, 2.500000000000002220, 1.029744260000002631 ) ;
#6742=CARTESIAN_POINT ( 'NONE',  ( 219.9999999999999716, -85.00000000000007105, 169.9999999999999716 ) ) ;
#6743=FACE_BOUND ( 'NONE', #190, .T. ) ;
#6746=DIRECTION ( 'NONE',  ( -0.000000000000000000, -0.000000000000000000, -1.000000000000000000 ) ) ;
#6749=ORIENTED_EDGE ( 'NONE', *, *, #2424, .F. ) ;
#6751=CARTESIAN_POINT ( 'NONE',  ( 140.0000000000000000, -95.00000000000008527, 190.0000000000000000 ) ) ;
#6754=ADVANCED_FACE ( 'NONE', ( #3228, #8581 ), #11929, .F. ) ;
#6756=VERTEX_POINT ( 'NONE', #9677 ) ;
#6758=ORIENTED_EDGE ( 'NONE', *, *, #434, .T. ) ;
#6764=DIRECTION ( 'NONE',  ( 0.000000000000000000, 0.000000000000000000, -1.000000000000000000 ) ) ;
#6768=EDGE_CURVE ( 'NONE', #8550, #10315, #868, .T. ) ;
#6769=LINE ( 'NONE', #2559, #366 ) ;
#6789=DIRECTION ( 'NONE',  ( -0.000000000000000000, -1.000000000000000000, -0.000000000000000000 ) ) ;
#6794=CARTESIAN_POINT ( 'NONE',  ( 307.5000000000000000, -56.99999999999997158, -180.0000000000000000 ) ) ;
#6797=EDGE_CURVE ( 'NONE', #3720, #3167, #4074, .T. ) ;
#6800=FACE_OUTER_BOUND ( 'NONE', #11265, .T. ) ;
#6802=ORIENTED_EDGE ( 'NONE', *, *, #6214, .F. ) ;
#6803=CARTESIAN_POINT ( 'NONE',  ( 136.6666666666666288, -20.00000000000000000, 225.1500000000000625 ) ) ;
#6804=PRODUCT_DEFINITION_SHAPE ( 'NONE', 'NONE',  #2142 ) ;
#6809=FACE_OUTER_BOUND ( 'NONE', #6615, .T. ) ;
#6811=CARTESIAN_POINT ( 'NONE',  ( 305.0000000000000000, -36.99999999999997868, -180.0000000000000000 ) ) ;
#6821=DIRECTION ( 'NONE',  ( -0.000000000000000000, -0.000000000000000000, -1.000000000000000000 ) ) ;
#6831=ADVANCED_FACE ( 'NONE', ( #2193 ), #6479, .F. ) ;
#6834=FACE_OUTER_BOUND ( 'NONE', #6129, .T. ) ;
#6844=ADVANCED_FACE ( 'NONE', ( #14092 ), #3008, .F. ) ;
#6845=AXIS2_PLACEMENT_3D ( 'NONE', #5193, #9822, #6406 ) ;
#6846=CARTESIAN_POINT ( 'NONE',  ( 219.9999999999999716, -20.00000000000000000, -219.8500000000001080 ) ) ;
#6847=VECTOR ( 'NONE', #9856, 1000.000000000000000 ) ;
#6851=CARTESIAN_POINT ( 'NONE',  ( 134.9999999999999432, -36.99999999999997868, -180.0000000000000000 ) ) ;
#6852=DIRECTION ( 'NONE',  ( -0.000000000000000000, 1.000000000000000000, -0.000000000000000000 ) ) ;
#6854=CIRCLE ( 'NONE', #6845, 2.649999999999985700 ) ;
#6855=DIRECTION ( 'NONE',  ( 1.000000000000000000, 0.000000000000000000, 0.000000000000000000 ) ) ;
#6859=EDGE_LOOP ( 'NONE', ( #12790, #12781, #7038, #12421, #4075, #9134, #6528, #9065, #10367, #10082, #1906, #9757 ) ) ;
#6860=CIRCLE ( 'NONE', #3610, 2.649999999999985700 ) ;
#6861=DIRECTION ( 'NONE',  ( 1.000000000000000000, 0.000000000000000000, 0.000000000000000000 ) ) ;
#6862=AXIS2_PLACEMENT_3D ( 'NONE', #12291, #5412, #3313 ) ;
#6865=VECTOR ( 'NONE', #12133, 1000.000000000000000 ) ;
#6868=LINE ( 'NONE', #13325, #2920 ) ;
#6872=AXIS2_PLACEMENT_3D ( 'NONE', #6901, #1451, #12557 ) ;
#6873=ORIENTED_EDGE ( 'NONE', *, *, #13953, .T. ) ;
#6877=CIRCLE ( 'NONE', #12219, 2.649999999999985700 ) ;
#6884=CYLINDRICAL_SURFACE ( 'NONE', #12950, 2.500000000000002220 ) ;
#6891=DIRECTION ( 'NONE',  ( -0.000000000000000000, -0.000000000000000000, -1.000000000000000000 ) ) ;
#6895=AXIS2_PLACEMENT_3D ( 'NONE', #6811, #44, #11313 ) ;
#6897=DIRECTION ( 'NONE',  ( 0.000000000000000000, 0.000000000000000000, 1.000000000000000000 ) ) ;
#6899=DIRECTION ( 'NONE',  ( -0.000000000000000000, -1.000000000000000000, -0.000000000000000000 ) ) ;
#6901=CARTESIAN_POINT ( 'NONE',  ( 140.0000000000000000, -75.00000000000008527, 190.0000000000000000 ) ) ;
#6905=CARTESIAN_POINT ( 'NONE',  ( 134.9999999999999432, -36.99999999999997868, -169.9999999999999716 ) ) ;
#6906=EDGE_LOOP ( 'NONE', ( #6201, #13009, #1132, #11532 ) ) ;
#6910=FACE_OUTER_BOUND ( 'NONE', #11822, .T. ) ;
#6913=VERTEX_POINT ( 'NONE', #10236 ) ;
#6921=CARTESIAN_POINT ( 'NONE',  ( 142.6500000000000057, -75.00000000000008527, -190.0000000000000000 ) ) ;
#6924=ADVANCED_FACE ( 'NONE', ( #8048 ), #1231, .F. ) ;
#6940=VERTEX_POINT ( 'NONE', #11255 ) ;
#6957=ORIENTED_EDGE ( 'NONE', *, *, #13180, .T. ) ;
#6960=DIRECTION ( 'NONE',  ( -0.000000000000000000, -0.000000000000000000, 1.000000000000000000 ) ) ;
#6961=CIRCLE ( 'NONE', #1629, 2.649999999999985700 ) ;
#6963=ORIENTED_EDGE ( 'NONE', *, *, #9972, .F. ) ;
#6965=EDGE_LOOP ( 'NONE', ( #9396, #1749, #7008 ) ) ;
#6968=AXIS2_PLACEMENT_3D ( 'NONE', #9390, #3876, #12435 ) ;
#6970=CARTESIAN_POINT ( 'NONE',  ( 136.6666666666666288, -25.00000000000000000, -225.1500000000000625 ) ) ;
#6971=ORIENTED_EDGE ( 'NONE', *, *, #1803, .F. ) ;
#6973=EDGE_CURVE ( 'NONE', #7848, #5316, #10164, .T. ) ;
#6983=VECTOR ( 'NONE', #10260, 1000.000000000000000 ) ;
#6993=DIRECTION ( 'NONE',  ( 1.000000000000000000, 0.000000000000000000, 0.000000000000000000 ) ) ;
#6997=EDGE_CURVE ( 'NONE', #12847, #8809, #7771, .T. ) ;
#6998=ORIENTED_EDGE ( 'NONE', *, *, #6614, .T. ) ;
#7000=( GEOMETRIC_REPRESENTATION_CONTEXT ( 3 ) GLOBAL_UNCERTAINTY_ASSIGNED_CONTEXT ( ( #14085 ) ) GLOBAL_UNIT_ASSIGNED_CONTEXT ( ( #5987, #439, #9327 ) ) REPRESENTATION_CONTEXT ( 'NONE', 'WORKASPACE' ) );
#7001=VECTOR ( 'NONE', #5320, 1000.000000000000000 ) ;
#7003=CARTESIAN_POINT ( 'NONE',  ( 299.9999999999999432, -75.00000000000008527, 190.0000000000000000 ) ) ;
#7007=ORIENTED_EDGE ( 'NONE', *, *, #14207, .F. ) ;
#7008=ORIENTED_EDGE ( 'NONE', *, *, #5092, .T. ) ;
#7010=FACE_OUTER_BOUND ( 'NONE', #4920, .T. ) ;
#7015=CARTESIAN_POINT ( 'NONE',  ( 299.9999999999999432, -95.00000000000008527, 190.0000000000000000 ) ) ;
#7017=ORIENTED_EDGE ( 'NONE', *, *, #3061, .F. ) ;
#7020=DIRECTION ( 'NONE',  ( -0.000000000000000000, -0.000000000000000000, -1.000000000000000000 ) ) ;
#7022=DIRECTION ( 'NONE',  ( 0.000000000000000000, 1.000000000000000000, 0.000000000000000000 ) ) ;
#7023=EDGE_CURVE ( 'NONE', #9740, #5927, #8461, .T. ) ;
#7026=CYLINDRICAL_SURFACE ( 'NONE', #1557, 2.649999999999985700 ) ;
#7029=CARTESIAN_POINT ( 'NONE',  ( 305.4999999999999432, -75.00000000000008527, -190.0000000000000000 ) ) ;
#7035=DIRECTION ( 'NONE',  ( -0.000000000000000000, -0.000000000000000000, 1.000000000000000000 ) ) ;
#7037=DIRECTION ( 'NONE',  ( 0.000000000000000000, 0.000000000000000000, 1.000000000000000000 ) ) ;
#7038=ORIENTED_EDGE ( 'NONE', *, *, #13435, .F. ) ;
#7039=CYLINDRICAL_SURFACE ( 'NONE', #8968, 2.649999999999985700 ) ;
#7049=FACE_OUTER_BOUND ( 'NONE', #12196, .T. ) ;
#7051=ORIENTED_EDGE ( 'NONE', *, *, #6144, .T. ) ;
#7061=AXIS2_PLACEMENT_3D ( 'NONE', #7691, #7759, #8649 ) ;
#7062=CARTESIAN_POINT ( 'NONE',  ( 53.33333333333330017, -20.00000000000000000, 225.1500000000000625 ) ) ;
#7063=AXIS2_PLACEMENT_3D ( 'NONE', #11217, #9028, #2578 ) ;
#7064=CARTESIAN_POINT ( 'NONE',  ( 140.0000000000000000, -95.00000000000008527, 190.0000000000000000 ) ) ;
#7065=CARTESIAN_POINT ( 'NONE',  ( -30.00000000000002842, -20.00000000000000000, 250.0000000000000000 ) ) ;
#7066=DIRECTION ( 'NONE',  ( -0.000000000000000000, -0.000000000000000000, -1.000000000000000000 ) ) ;
#7079=ORIENTED_EDGE ( 'NONE', *, *, #704, .T. ) ;
#7083=FACE_BOUND ( 'NONE', #7493, .T. ) ;
#7084=ADVANCED_FACE ( 'NONE', ( #1584 ), #11610, .F. ) ;
#7085=CIRCLE ( 'NONE', #5973, 5.500000000000005329 ) ;
#7087=EDGE_CURVE ( 'NONE', #2907, #13843, #3391, .T. ) ;
#7090=DIRECTION ( 'NONE',  ( 0.000000000000000000, 1.000000000000000000, 0.000000000000000000 ) ) ;
#7096=VECTOR ( 'NONE', #7022, 1000.000000000000000 ) ;
#7108=ORIENTED_EDGE ( 'NONE', *, *, #13504, .F. ) ;
#7110=ADVANCED_FACE ( 'NONE', ( #3996 ), #1449, .F. ) ;
#7119=DIRECTION ( 'NONE',  ( 0.000000000000000000, 0.000000000000000000, 1.000000000000000000 ) ) ;
#7127=ORIENTED_EDGE ( 'NONE', *, *, #7366, .F. ) ;
#7137=FACE_BOUND ( 'NONE', #13938, .T. ) ;
#7138=CARTESIAN_POINT ( 'NONE',  ( 134.9999999999999432, -56.99999999999997158, -180.0000000000000000 ) ) ;
#7139=DIRECTION ( 'NONE',  ( -0.000000000000000000, -0.000000000000000000, -1.000000000000000000 ) ) ;
#7140=DIRECTION ( 'NONE',  ( -0.000000000000000000, -0.000000000000000000, 1.000000000000000000 ) ) ;
#7141=EDGE_LOOP ( 'NONE', ( #14199, #9842, #10248, #11411 ) ) ;
#7149=DIRECTION ( 'NONE',  ( 1.000000000000000000, 0.000000000000000000, 0.000000000000000000 ) ) ;
#7150=EDGE_CURVE ( 'NONE', #5386, #4689, #9439, .T. ) ;
#7156=CARTESIAN_POINT ( 'NONE',  ( 219.9999999999999716, -25.00000000000000000, -222.5000000000000853 ) ) ;
#7168=ADVANCED_FACE ( 'NONE', ( #13853 ), #11400, .F. ) ;
#7172=DIRECTION ( 'NONE',  ( -1.000000000000000000, 0.000000000000000000, 0.000000000000000000 ) ) ;
#7173=CARTESIAN_POINT ( 'NONE',  ( 137.3500000000000227, -75.00000000000008527, -169.9999999999999716 ) ) ;
#7176=CARTESIAN_POINT ( 'NONE',  ( 140.0000000000000000, -95.00000000000008527, -169.9999999999999716 ) ) ;
#7177=EDGE_LOOP ( 'NONE', ( #1096, #5732, #9899, #10046 ) ) ;
#7178=AXIS2_PLACEMENT_3D ( 'NONE', #8476, #12908, #7395 ) ;
#7181=ORIENTED_EDGE ( 'NONE', *, *, #12098, .F. ) ;
#7185=AXIS2_PLACEMENT_3D ( 'NONE', #8843, #9048, #13266 ) ;
#7187=AXIS2_PLACEMENT_3D ( 'NONE', #13647, #9309, #3719 ) ;
#7193=DIRECTION ( 'NONE',  ( -0.000000000000000000, -0.000000000000000000, -1.000000000000000000 ) ) ;
#7204=EDGE_CURVE ( 'NONE', #5871, #14256, #6387, .T. ) ;
#7206=EDGE_CURVE ( 'NONE', #14256, #8359, #12878, .T. ) ;
#7208=VECTOR ( 'NONE', #5835, 1000.000000000000000 ) ;
#7209=DIRECTION ( 'NONE',  ( 1.000000000000000000, 0.000000000000000000, 0.000000000000000000 ) ) ;
#7214=DIRECTION ( 'NONE',  ( -0.000000000000000000, 1.000000000000000000, -0.000000000000000000 ) ) ;
#7218=CARTESIAN_POINT ( 'NONE',  ( 303.3333333333333144, -25.00000000000000000, -222.5000000000000853 ) ) ;
#7230=CARTESIAN_POINT ( 'NONE',  ( 140.0000000000000000, -95.00000000000008527, -169.9999999999999716 ) ) ;
#7236=ORIENTED_EDGE ( 'NONE', *, *, #14113, .F. ) ;
#7242=DIRECTION ( 'NONE',  ( -0.000000000000000000, -0.000000000000000000, -1.000000000000000000 ) ) ;
#7251=CARTESIAN_POINT ( 'NONE',  ( 299.9999999999999432, -95.00000000000008527, -190.0000000000000000 ) ) ;
#7257=CARTESIAN_POINT ( 'NONE',  ( 140.0000000000000000, -95.00000000000008527, -186.2999999999999829 ) ) ;
#7259=EDGE_CURVE ( 'NONE', #6389, #9136, #336, .T. ) ;
#7260=CARTESIAN_POINT ( 'NONE',  ( 303.3333333333333144, -20.00000000000000000, -225.1500000000000625 ) ) ;
#7263=DIRECTION ( 'NONE',  ( 0.000000000000000000, 0.000000000000000000, 1.000000000000000000 ) ) ;
#7265=VERTEX_POINT ( 'NONE', #14134 ) ;
#7270=ORIENTED_EDGE ( 'NONE', *, *, #8842, .T. ) ;
#7272=ORIENTED_EDGE ( 'NONE', *, *, #7868, .T. ) ;
#7274=DIRECTION ( 'NONE',  ( -0.000000000000000000, -0.000000000000000000, 1.000000000000000000 ) ) ;
#7275=PLANE ( 'NONE',  #2234 ) ;
#7276=EDGE_CURVE ( 'NONE', #6389, #10563, #5169, .T. ) ;
#7282=ORIENTED_EDGE ( 'NONE', *, *, #878, .F. ) ;
#7290=FACE_BOUND ( 'NONE', #11732, .T. ) ;
#7291=VERTEX_POINT ( 'NONE', #7400 ) ;
#7303=DIRECTION ( 'NONE',  ( 0.000000000000000000, -1.000000000000000000, 0.000000000000000000 ) ) ;
#7306=CARTESIAN_POINT ( 'NONE',  ( 201.0000000000000000, -85.00000000000007105, 190.0000000000000000 ) ) ;
#7311=EDGE_LOOP ( 'NONE', ( #1203, #10944, #5188, #7515 ) ) ;
#7312=CARTESIAN_POINT ( 'NONE',  ( 302.6499999999999204, -75.00000000000008527, -186.2999999999999829 ) ) ;
#7314=ORIENTED_EDGE ( 'NONE', *, *, #7513, .T. ) ;
#7320=CARTESIAN_POINT ( 'NONE',  ( 132.4999999999999432, -36.99999999999997868, -169.9999999999999716 ) ) ;
#7322=DIRECTION ( 'NONE',  ( -1.000000000000000000, 0.000000000000000000, 0.000000000000000000 ) ) ;
#7324=VERTEX_POINT ( 'NONE', #5789 ) ;
#7332=PLANE ( 'NONE',  #10133 ) ;
#7333=VERTEX_POINT ( 'NONE', #5650 ) ;
#7339=CIRCLE ( 'NONE', #1066, 2.649999999999985700 ) ;
#7346=CARTESIAN_POINT ( 'NONE',  ( 53.33333333333330017, -25.00000000000000000, 225.1500000000000625 ) ) ;
#7354=VECTOR ( 'NONE', #8004, 1000.000000000000000 ) ;
#7357=EDGE_CURVE ( 'NONE', #11325, #5316, #5255, .T. ) ;
#7363=EDGE_LOOP ( 'NONE', ( #10665, #699, #13887, #3842 ) ) ;
#7366=EDGE_CURVE ( 'NONE', #7265, #5572, #2452, .T. ) ;
#7371=EDGE_LOOP ( 'NONE', ( #11026, #13611, #6670, #10101 ) ) ;
#7376=DIRECTION ( 'NONE',  ( 1.000000000000000000, 0.000000000000000000, 0.000000000000000000 ) ) ;
#7377=ORIENTED_EDGE ( 'NONE', *, *, #3174, .T. ) ;
#7382=EDGE_CURVE ( 'NONE', #13697, #11046, #113, .T. ) ;
#7383=LINE ( 'NONE', #13906, #3503 ) ;
#7391=ADVANCED_FACE ( 'NONE', ( #6809 ), #2387, .F. ) ;
#7392=DIRECTION ( 'NONE',  ( 0.000000000000000000, 0.000000000000000000, -1.000000000000000000 ) ) ;
#7395=DIRECTION ( 'NONE',  ( 1.000000000000000000, 0.000000000000000000, 0.000000000000000000 ) ) ;
#7400=CARTESIAN_POINT ( 'NONE',  ( 136.6666666666666288, -20.00000000000000000, -225.1500000000000625 ) ) ;
#7404=CARTESIAN_POINT ( 'NONE',  ( 119.9999999999999147, -225.0010000000000048, -19.99999999999998934 ) ) ;
#7409=CARTESIAN_POINT ( 'NONE',  ( 119.9999999999999147, -20.00000000000000000, 169.9999999999999716 ) ) ;
#7410=CARTESIAN_POINT ( 'NONE',  ( 53.33333333333330017, -25.00000000000000000, 222.5000000000000853 ) ) ;
#7416=VECTOR ( 'NONE', #6383, 1000.000000000000000 ) ;
#7424=DIRECTION ( 'NONE',  ( 1.000000000000000000, 0.000000000000000000, 0.000000000000000000 ) ) ;
#7427=VECTOR ( 'NONE', #7193, 1000.000000000000000 ) ;
#7432=CARTESIAN_POINT ( 'NONE',  ( 294.4999999999999432, -95.00000000000008527, -190.0000000000000000 ) ) ;
#7433=ADVANCED_FACE ( 'NONE', ( #8985 ), #10072, .F. ) ;
#7438=FACE_BOUND ( 'NONE', #7464, .T. ) ;
#7447=ORIENTED_EDGE ( 'NONE', *, *, #4743, .T. ) ;
#7453=ORIENTED_EDGE ( 'NONE', *, *, #11718, .F. ) ;
#7456=EDGE_CURVE ( 'NONE', #10523, #11569, #7814, .T. ) ;
#7457=DIRECTION ( 'NONE',  ( -0.000000000000000000, 1.000000000000000000, -0.000000000000000000 ) ) ;
#7463=STYLED_ITEM ( 'NONE', ( #4454 ), #12845 ) ;
#7464=EDGE_LOOP ( 'NONE', ( #11606, #211 ) ) ;
#7466=FACE_OUTER_BOUND ( 'NONE', #14153, .T. ) ;
#7467=DIRECTION ( 'NONE',  ( -0.000000000000000000, -0.000000000000000000, -1.000000000000000000 ) ) ;
#7470=EDGE_LOOP ( 'NONE', ( #2291, #3518, #912, #1230 ) ) ;
#7472=DIRECTION ( 'NONE',  ( 1.000000000000000000, 0.000000000000000000, 0.000000000000000000 ) ) ;
#7479=ORIENTED_EDGE ( 'NONE', *, *, #3733, .T. ) ;
#7484=EDGE_LOOP ( 'NONE', ( #4232, #13643 ) ) ;
#7487=AXIS2_PLACEMENT_3D ( 'NONE', #12110, #2169, #10668 ) ;
#7490=EDGE_LOOP ( 'NONE', ( #857, #11543, #7532, #5783 ) ) ;
#7492=CARTESIAN_POINT ( 'NONE',  ( 386.6666666666666288, -20.00000000000000000, 222.5000000000000853 ) ) ;
#7493=EDGE_LOOP ( 'NONE', ( #3718, #10640 ) ) ;
#7507=LINE ( 'NONE', #2067, #380 ) ;
#7510=CARTESIAN_POINT ( 'NONE',  ( 303.3333333333333144, -20.00000000000000000, -222.5000000000000853 ) ) ;
#7513=EDGE_CURVE ( 'NONE', #10689, #5572, #6860, .T. ) ;
#7515=ORIENTED_EDGE ( 'NONE', *, *, #6688, .F. ) ;
#7521=DIRECTION ( 'NONE',  ( -0.000000000000000000, 1.000000000000000000, -0.000000000000000000 ) ) ;
#7523=DIRECTION ( 'NONE',  ( -1.000000000000000000, 0.000000000000000000, 0.000000000000000000 ) ) ;
#7528=DIRECTION ( 'NONE',  ( -1.000000000000000000, 0.000000000000000000, 0.000000000000000000 ) ) ;
#7531=ADVANCED_FACE ( 'NONE', ( #13613, #1714, #9126, #7083, #1563, #13828 ), #13532, .F. ) ;
#7532=ORIENTED_EDGE ( 'NONE', *, *, #9415, .T. ) ;
#7538=FACE_BOUND ( 'NONE', #1422, .T. ) ;
#7541=ADVANCED_FACE ( 'NONE', ( #2530 ), #11378, .F. ) ;
#7543=AXIS2_PLACEMENT_3D ( 'NONE', #9887, #3084, #7424 ) ;
#7548=DIRECTION ( 'NONE',  ( -0.000000000000000000, -1.000000000000000000, -0.000000000000000000 ) ) ;
#7564=CONICAL_SURFACE ( 'NONE', #10336, 2.500000000000002220, 1.029744260000002631 ) ;
#7566=EDGE_CURVE ( 'NONE', #1448, #12847, #11665, .T. ) ;
#7568=EDGE_LOOP ( 'NONE', ( #9929, #3649 ) ) ;
#7571=AXIS2_PLACEMENT_3D ( 'NONE', #9531, #11852, #12791 ) ;
#7572=CARTESIAN_POINT ( 'NONE',  ( 302.6499999999999204, -75.00000000000008527, -186.2999999999999829 ) ) ;
#7573=ORIENTED_EDGE ( 'NONE', *, *, #13026, .T. ) ;
#7576=DIRECTION ( 'NONE',  ( -0.000000000000000000, 0.000000000000000000, 1.000000000000000000 ) ) ;
#7581=DIRECTION ( 'NONE',  ( -1.000000000000000000, 0.000000000000000000, 0.000000000000000000 ) ) ;
#7583=CARTESIAN_POINT ( 'NONE',  ( 134.9999999999999432, -36.99999999999997868, -180.0000000000000000 ) ) ;
#7589=VERTEX_POINT ( 'NONE', #12746 ) ;
#7597=CIRCLE ( 'NONE', #11193, 2.649999999999985700 ) ;
#7600=VERTEX_POINT ( 'NONE', #12599 ) ;
#7601=LINE ( 'NONE', #4209, #11628 ) ;
#7605=ORIENTED_EDGE ( 'NONE', *, *, #3477, .T. ) ;
#7608=ORIENTED_EDGE ( 'NONE', *, *, #12859, .F. ) ;
#7615=EDGE_CURVE ( 'NONE', #2215, #6940, #4196, .T. ) ;
#7621=DIRECTION ( 'NONE',  ( -1.000000000000000000, 0.000000000000000000, 0.000000000000000000 ) ) ;
#7622=ORIENTED_EDGE ( 'NONE', *, *, #6614, .F. ) ;
#7624=CIRCLE ( 'NONE', #5321, 5.500000000000005329 ) ;
#7626=ORIENTED_EDGE ( 'NONE', *, *, #12517, .T. ) ;
#7630=CARTESIAN_POINT ( 'NONE',  ( 140.0000000000000000, -75.00000000000008527, 190.0000000000000000 ) ) ;
#7634=AXIS2_PLACEMENT_3D ( 'NONE', #7583, #2212, #5631 ) ;
#7637=DIRECTION ( 'NONE',  ( -0.000000000000000000, -1.000000000000000000, -0.000000000000000000 ) ) ;
#7639=VERTEX_POINT ( 'NONE', #11888 ) ;
#7640=VECTOR ( 'NONE', #525, 1000.000000000000000 ) ;
#7646=ADVANCED_FACE ( 'NONE', ( #12892 ), #11956, .F. ) ;
#7651=ADVANCED_FACE ( 'NONE', ( #13101 ), #899, .F. ) ;
#7653=AXIS2_PLACEMENT_3D ( 'NONE', #4645, #3486, #7954 ) ;
#7662=DIRECTION ( 'NONE',  ( -0.000000000000000000, -0.000000000000000000, 1.000000000000000000 ) ) ;
#7663=AXIS2_PLACEMENT_3D ( 'NONE', #5988, #2650, #4693 ) ;
#7664=LINE ( 'NONE', #12101, #13186 ) ;
#7671=ORIENTED_EDGE ( 'NONE', *, *, #7206, .T. ) ;
#7672=DIRECTION ( 'NONE',  ( -0.8571673013836870192, 1.049727191973306873E-16, 0.5150380737757234151 ) ) ;
#7673=PLANE ( 'NONE',  #3026 ) ;
#7691=CARTESIAN_POINT ( 'NONE',  ( 236.4999999999999432, -85.00000000000007105, 180.0000000000000000 ) ) ;
#7692=ORIENTED_EDGE ( 'NONE', *, *, #8451, .F. ) ;
#7696=ORIENTED_EDGE ( 'NONE', *, *, #5243, .T. ) ;
#7698=VERTEX_POINT ( 'NONE', #14119 ) ;
#7700=CARTESIAN_POINT ( 'NONE',  ( 203.5000000000000000, -85.00000000000007105, 190.0000000000000000 ) ) ;
#7704=AXIS2_PLACEMENT_3D ( 'NONE', #3562, #11534, #9363 ) ;
#7705=FACE_OUTER_BOUND ( 'NONE', #1407, .T. ) ;
#7715=DIRECTION ( 'NONE',  ( -1.000000000000000000, 0.000000000000000000, 0.000000000000000000 ) ) ;
#7728=ORIENTED_EDGE ( 'NONE', *, *, #2055, .T. ) ;
#7729=CARTESIAN_POINT ( 'NONE',  ( 142.6500000000000057, -75.00000000000008527, -186.2999999999999829 ) ) ;
#7735=DIRECTION ( 'NONE',  ( -0.000000000000000000, -0.000000000000000000, -1.000000000000000000 ) ) ;
#7737=DIRECTION ( 'NONE',  ( -0.000000000000000000, -0.000000000000000000, 1.000000000000000000 ) ) ;
#7743=ORIENTED_EDGE ( 'NONE', *, *, #8229, .F. ) ;
#7750=DIRECTION ( 'NONE',  ( -0.000000000000000000, -0.000000000000000000, 1.000000000000000000 ) ) ;
#7751=LINE ( 'NONE', #45, #8306 ) ;
#7753=CARTESIAN_POINT ( 'NONE',  ( 319.9999999999999432, -20.00000000000000000, -19.99999999999998934 ) ) ;
#7757=ORIENTED_EDGE ( 'NONE', *, *, #8640, .T. ) ;
#7759=DIRECTION ( 'NONE',  ( -0.000000000000000000, -0.000000000000000000, 1.000000000000000000 ) ) ;
#7760=AXIS2_PLACEMENT_3D ( 'NONE', #7312, #9360, #13770 ) ;
#7762=CARTESIAN_POINT ( 'NONE',  ( 299.9999999999999432, -95.00000000000008527, -190.0000000000000000 ) ) ;
#7765=ORIENTED_EDGE ( 'NONE', *, *, #9443, .T. ) ;
#7767=CARTESIAN_POINT ( 'NONE',  ( 305.4999999999999432, -95.00000000000008527, 190.0000000000000000 ) ) ;
#7769=ADVANCED_FACE ( 'NONE', ( #8883 ), #3660, .F. ) ;
#7771=CIRCLE ( 'NONE', #322, 2.649999999999985700 ) ;
#7782=DIRECTION ( 'NONE',  ( -0.000000000000000000, -0.000000000000000000, -1.000000000000000000 ) ) ;
#7788=DIRECTION ( 'NONE',  ( -0.000000000000000000, 1.000000000000000000, -0.000000000000000000 ) ) ;
#7800=DIRECTION ( 'NONE',  ( -0.000000000000000000, -0.000000000000000000, 1.000000000000000000 ) ) ;
#7811=FACE_OUTER_BOUND ( 'NONE', #11235, .T. ) ;
#7812=ORIENTED_EDGE ( 'NONE', *, *, #13849, .T. ) ;
#7814=LINE ( 'NONE', #12253, #10808 ) ;
#7815=EDGE_CURVE ( 'NONE', #14007, #2814, #1118, .T. ) ;
#7825=CARTESIAN_POINT ( 'NONE',  ( 134.9999999999999432, -36.99999999999997868, -180.0000000000000000 ) ) ;
#7830=ORIENTED_EDGE ( 'NONE', *, *, #6336, .T. ) ;
#7840=DIRECTION ( 'NONE',  ( -1.000000000000000000, 0.000000000000000000, 0.000000000000000000 ) ) ;
#7842=CARTESIAN_POINT ( 'NONE',  ( 305.4999999999999432, -75.00000000000008527, 190.0000000000000000 ) ) ;
#7845=FACE_BOUND ( 'NONE', #320, .T. ) ;
#7848=VERTEX_POINT ( 'NONE', #5491 ) ;
#7853=CARTESIAN_POINT ( 'NONE',  ( -30.00000000000002842, -25.00000000000000000, -169.9999999999999716 ) ) ;
#7854=DIRECTION ( 'NONE',  ( 1.000000000000000000, 0.000000000000000000, 0.000000000000000000 ) ) ;
#7859=CARTESIAN_POINT ( 'NONE',  ( 136.6666666666666288, -25.00000000000000000, -222.5000000000000853 ) ) ;
#7861=VERTEX_POINT ( 'NONE', #1195 ) ;
#7867=EDGE_LOOP ( 'NONE', ( #10468, #5166, #13279, #8632 ) ) ;
#7868=EDGE_CURVE ( 'NONE', #9652, #4280, #10590, .T. ) ;
#7873=AXIS2_PLACEMENT_3D ( 'NONE', #14052, #7457, #11892 ) ;
#7875=LINE ( 'NONE', #5574, #12175 ) ;
#7878=VECTOR ( 'NONE', #1622, 1000.000000000000000 ) ;
#7880=ORIENTED_EDGE ( 'NONE', *, *, #3434, .T. ) ;
#7884=CARTESIAN_POINT ( 'NONE',  ( 236.4999999999999432, -85.00000000000007105, 180.0000000000000000 ) ) ;
#7889=DIRECTION ( 'NONE',  ( -0.000000000000000000, -0.000000000000000000, 1.000000000000000000 ) ) ;
#7891=VECTOR ( 'NONE', #11141, 1000.000000000000000 ) ;
#7894=EDGE_CURVE ( 'NONE', #12590, #1452, #2941, .T. ) ;
#7895=EDGE_CURVE ( 'NONE', #3696, #11791, #2159, .T. ) ;
#7896=DIRECTION ( 'NONE',  ( 1.000000000000000000, 0.000000000000000000, 0.000000000000000000 ) ) ;
#7898=ADVANCED_FACE ( 'NONE', ( #10474 ), #4095, .F. ) ;
#7900=EDGE_LOOP ( 'NONE', ( #10516, #2829, #6706, #11124 ) ) ;
#7904=CARTESIAN_POINT ( 'NONE',  ( 294.4999999999999432, -75.00000000000008527, 186.2999999999999829 ) ) ;
#7910=SURFACE_STYLE_FILL_AREA ( #6623 ) ;
#7929=ORIENTED_EDGE ( 'NONE', *, *, #8902, .T. ) ;
#7932=CARTESIAN_POINT ( 'NONE',  ( 299.9999999999999432, -95.00000000000008527, -190.0000000000000000 ) ) ;
#7934=CIRCLE ( 'NONE', #7487, 5.500000000000005329 ) ;
#7938=ORIENTED_EDGE ( 'NONE', *, *, #8445, .F. ) ;
#7939=DIRECTION ( 'NONE',  ( 1.000000000000000000, 0.000000000000000000, 0.000000000000000000 ) ) ;
#7940=ADVANCED_FACE ( 'NONE', ( #3872 ), #7275, .F. ) ;
#7943=EDGE_LOOP ( 'NONE', ( #7272, #12957 ) ) ;
#7945=DIRECTION ( 'NONE',  ( -0.000000000000000000, -0.000000000000000000, 1.000000000000000000 ) ) ;
#7954=DIRECTION ( 'NONE',  ( -1.000000000000000000, 0.000000000000000000, 0.000000000000000000 ) ) ;
#7955=CARTESIAN_POINT ( 'NONE',  ( 137.4999999999999432, -36.99999999999997868, -169.9999999999999716 ) ) ;
#7961=ADVANCED_FACE ( 'NONE', ( #7137, #9537, #2716, #1753, #6192, #657 ), #1686, .F. ) ;
#7963=EDGE_CURVE ( 'NONE', #1839, #12345, #10546, .T. ) ;
#7974=CARTESIAN_POINT ( 'NONE',  ( 470.0000000000000000, -25.00000000000000000, 250.0000000000000000 ) ) ;
#7975=FILL_AREA_STYLE_COLOUR ( '', #13713 ) ;
#7977=CYLINDRICAL_SURFACE ( 'NONE', #8511, 2.500000000000002220 ) ;
#7978=ORIENTED_EDGE ( 'NONE', *, *, #12352, .F. ) ;
#7981=ORIENTED_EDGE ( 'NONE', *, *, #1323, .F. ) ;
#7986=VERTEX_POINT ( 'NONE', #12720 ) ;
#7989=CARTESIAN_POINT ( 'NONE',  ( 319.9999999999999432, -225.0010000000000048, 169.9999999999999716 ) ) ;
#7995=DIRECTION ( 'NONE',  ( 1.000000000000000000, 0.000000000000000000, 0.000000000000000000 ) ) ;
#8002=CYLINDRICAL_SURFACE ( 'NONE', #12525, 2.649999999999985700 ) ;
#8004=DIRECTION ( 'NONE',  ( -0.000000000000000000, -0.000000000000000000, -1.000000000000000000 ) ) ;
#8008=CARTESIAN_POINT ( 'NONE',  ( 299.9999999999999432, -75.00000000000008527, -190.0000000000000000 ) ) ;
#8009=AXIS2_PLACEMENT_3D ( 'NONE', #10995, #3242, #7715 ) ;
#8019=CARTESIAN_POINT ( 'NONE',  ( 386.6666666666666288, -20.00000000000000000, 219.8500000000001080 ) ) ;
#8020=CIRCLE ( 'NONE', #7571, 2.649999999999985700 ) ;
#8024=DIRECTION ( 'NONE',  ( -1.000000000000000000, 0.000000000000000000, 0.000000000000000000 ) ) ;
#8031=DIRECTION ( 'NONE',  ( -0.000000000000000000, -0.000000000000000000, 1.000000000000000000 ) ) ;
#8040=DIRECTION ( 'NONE',  ( 0.000000000000000000, 1.000000000000000000, 0.000000000000000000 ) ) ;
#8041=EDGE_CURVE ( 'NONE', #4959, #8189, #1910, .T. ) ;
#8045=ORIENTED_EDGE ( 'NONE', *, *, #2918, .F. ) ;
#8046=DIRECTION ( 'NONE',  ( 0.000000000000000000, 1.000000000000000000, 0.000000000000000000 ) ) ;
#8048=FACE_OUTER_BOUND ( 'NONE', #11101, .T. ) ;
#8053=DIRECTION ( 'NONE',  ( -0.000000000000000000, 1.000000000000000000, -0.000000000000000000 ) ) ;
#8057=CARTESIAN_POINT ( 'NONE',  ( 469.9999999999998863, -225.0000000000000000, -169.9999999999999716 ) ) ;
#8059=VECTOR ( 'NONE', #10323, 1000.000000000000000 ) ;
#8071=EDGE_CURVE ( 'NONE', #7639, #10296, #11999, .T. ) ;
#8074=AXIS2_PLACEMENT_3D ( 'NONE', #5155, #12899, #7523 ) ;
#8075=CARTESIAN_POINT ( 'NONE',  ( 305.0000000000000000, -56.99999999999997158, -180.0000000000000000 ) ) ;
#8080=EDGE_CURVE ( 'NONE', #14219, #13531, #6428, .T. ) ;
#8085=ORIENTED_EDGE ( 'NONE', *, *, #1597, .F. ) ;
#8092=AXIS2_PLACEMENT_3D ( 'NONE', #9347, #2743, #4850 ) ;
#8094=VERTEX_POINT ( 'NONE', #3231 ) ;
#8097=CARTESIAN_POINT ( 'NONE',  ( 469.9999999999998863, -225.0000000000000000, -169.9999999999999716 ) ) ;
#8099=VERTEX_POINT ( 'NONE', #798 ) ;
#8102=DIRECTION ( 'NONE',  ( 0.000000000000000000, 0.000000000000000000, -1.000000000000000000 ) ) ;
#8108=CIRCLE ( 'NONE', #680, 10.00000000000000888 ) ;
#8114=VECTOR ( 'NONE', #8682, 1000.000000000000000 ) ;
#8117=ORIENTED_EDGE ( 'NONE', *, *, #10763, .T. ) ;
#8120=DIRECTION ( 'NONE',  ( 1.000000000000000000, 0.000000000000000000, 0.000000000000000000 ) ) ;
#8122=ORIENTED_EDGE ( 'NONE', *, *, #13322, .F. ) ;
#8128=FACE_BOUND ( 'NONE', #1023, .T. ) ;
#8130=CIRCLE ( 'NONE', #8365, 2.649999999999985700 ) ;
#8132=ORIENTED_EDGE ( 'NONE', *, *, #11575, .T. ) ;
#8133=DIRECTION ( 'NONE',  ( -0.8571673013836870192, 1.049727191973306873E-16, 0.5150380737757234151 ) ) ;
#8140=LINE ( 'NONE', #2499, #8059 ) ;
#8157=VERTEX_POINT ( 'NONE', #8728 ) ;
#8161=EDGE_CURVE ( 'NONE', #12143, #11802, #10770, .T. ) ;
#8162=CARTESIAN_POINT ( 'NONE',  ( 136.6666666666666288, -20.00000000000000000, -222.5000000000000853 ) ) ;
#8166=EDGE_LOOP ( 'NONE', ( #8862, #5787, #11870, #1550 ) ) ;
#8175=CARTESIAN_POINT ( 'NONE',  ( 134.5000000000000000, -75.00000000000008527, -186.2999999999999829 ) ) ;
#8188=CARTESIAN_POINT ( 'NONE',  ( 219.9999999999999716, -20.00000000000000000, -222.5000000000000853 ) ) ;
#8189=VERTEX_POINT ( 'NONE', #3638 ) ;
#8199=CARTESIAN_POINT ( 'NONE',  ( 236.4999999999999432, -85.00000000000007105, 190.0000000000000000 ) ) ;
#8200=ORIENTED_EDGE ( 'NONE', *, *, #2773, .F. ) ;
#8208=CARTESIAN_POINT ( 'NONE',  ( 203.5000000000000000, -85.00000000000007105, 178.4978484569338946 ) ) ;
#8214=DIRECTION ( 'NONE',  ( -0.000000000000000000, -0.000000000000000000, 1.000000000000000000 ) ) ;
#8218=CIRCLE ( 'NONE', #5684, 5.500000000000005329 ) ;
#8219=ORIENTED_EDGE ( 'NONE', *, *, #2946, .F. ) ;
#8224=DIRECTION ( 'NONE',  ( -0.000000000000000000, -0.000000000000000000, 1.000000000000000000 ) ) ;
#8229=EDGE_CURVE ( 'NONE', #13282, #4602, #7339, .T. ) ;
#8234=DIRECTION ( 'NONE',  ( -1.000000000000000000, 0.000000000000000000, 0.000000000000000000 ) ) ;
#8236=VERTEX_POINT ( 'NONE', #13424 ) ;
#8237=DIRECTION ( 'NONE',  ( 0.000000000000000000, 1.000000000000000000, 0.000000000000000000 ) ) ;
#8238=VECTOR ( 'NONE', #9618, 1000.000000000000000 ) ;
#8245=DIRECTION ( 'NONE',  ( -0.000000000000000000, -0.000000000000000000, -1.000000000000000000 ) ) ;
#8248=AXIS2_PLACEMENT_3D ( 'NONE', #6536, #2321, #4505 ) ;
#8249=CARTESIAN_POINT ( 'NONE',  ( 294.4999999999999432, -95.00000000000008527, 190.0000000000000000 ) ) ;
#8250=CIRCLE ( 'NONE', #3661, 2.649999999999985700 ) ;
#8252=ORIENTED_EDGE ( 'NONE', *, *, #12098, .T. ) ;
#8253=CIRCLE ( 'NONE', #2724, 5.500000000000005329 ) ;
#8263=CARTESIAN_POINT ( 'NONE',  ( 386.6666666666666288, -20.00000000000000000, -219.8500000000001080 ) ) ;
#8264=ORIENTED_EDGE ( 'NONE', *, *, #11466, .T. ) ;
#8266=CARTESIAN_POINT ( 'NONE',  ( 219.9999999999999716, -20.00000000000000000, -222.5000000000000853 ) ) ;
#8273=CARTESIAN_POINT ( 'NONE',  ( 299.9999999999999432, -75.00000000000008527, 190.0000000000000000 ) ) ;
#8281=ORIENTED_EDGE ( 'NONE', *, *, #871, .F. ) ;
#8287=ORIENTED_EDGE ( 'NONE', *, *, #11448, .T. ) ;
#8294=CARTESIAN_POINT ( 'NONE',  ( 303.3333333333333144, -25.00000000000000000, 225.1500000000000625 ) ) ;
#8305=CARTESIAN_POINT ( 'NONE',  ( 299.9999999999999432, -75.00000000000008527, 169.9999999999999716 ) ) ;
#8306=VECTOR ( 'NONE', #12258, 1000.000000000000000 ) ;
#8307=DIRECTION ( 'NONE',  ( -0.000000000000000000, -0.000000000000000000, 1.000000000000000000 ) ) ;
#8309=CARTESIAN_POINT ( 'NONE',  ( 137.3500000000000227, -95.00000000000008527, 169.9999999999999716 ) ) ;
#8310=DIRECTION ( 'NONE',  ( 0.000000000000000000, 1.000000000000000000, 0.000000000000000000 ) ) ;
#8312=ORIENTED_EDGE ( 'NONE', *, *, #13953, .F. ) ;
#8324=CARTESIAN_POINT ( 'NONE',  ( 469.9999999999998863, -225.0000000000000000, -169.9999999999999716 ) ) ;
#8328=FACE_OUTER_BOUND ( 'NONE', #6684, .T. ) ;
#8339=LINE ( 'NONE', #6168, #12920 ) ;
#8342=VECTOR ( 'NONE', #6712, 1000.000000000000000 ) ;
#8351=ADVANCED_FACE ( 'NONE', ( #6028 ), #8413, .F. ) ;
#8355=VECTOR ( 'NONE', #11352, 1000.000000000000000 ) ;
#8359=VERTEX_POINT ( 'NONE', #3999 ) ;
#8360=DIRECTION ( 'NONE',  ( -0.000000000000000000, -0.000000000000000000, -1.000000000000000000 ) ) ;
#8365=AXIS2_PLACEMENT_3D ( 'NONE', #412, #12700, #2771 ) ;
#8369=ORIENTED_EDGE ( 'NONE', *, *, #9018, .F. ) ;
#8376=CARTESIAN_POINT ( 'NONE',  ( 209.9999999999999716, -85.00000000000007105, 190.0000000000000000 ) ) ;
#8378=AXIS2_PLACEMENT_3D ( 'NONE', #9871, #8852, #11638 ) ;
#8379=DIRECTION ( 'NONE',  ( -0.000000000000000000, -0.000000000000000000, 1.000000000000000000 ) ) ;
#8387=VECTOR ( 'NONE', #8245, 1000.000000000000000 ) ;
#8404=ORIENTED_EDGE ( 'NONE', *, *, #2992, .F. ) ;
#8409=ORIENTED_EDGE ( 'NONE', *, *, #11917, .F. ) ;
#8413=CYLINDRICAL_SURFACE ( 'NONE', #9900, 5.500000000000005329 ) ;
#8416=EDGE_CURVE ( 'NONE', #6238, #2872, #12698, .T. ) ;
#8427=ORIENTED_EDGE ( 'NONE', *, *, #2929, .F. ) ;
#8429=ADVANCED_FACE ( 'NONE', ( #11686, #409, #4880, #14137, #2177 ), #4144, .F. ) ;
#8431=DIRECTION ( 'NONE',  ( -0.000000000000000000, -0.000000000000000000, 1.000000000000000000 ) ) ;
#8435=EDGE_CURVE ( 'NONE', #3125, #13571, #9910, .T. ) ;
#8437=ORIENTED_EDGE ( 'NONE', *, *, #5281, .F. ) ;
#8440=LINE ( 'NONE', #5336, #969 ) ;
#8445=EDGE_CURVE ( 'NONE', #2036, #11751, #6462, .T. ) ;
#8450=FACE_OUTER_BOUND ( 'NONE', #8774, .T. ) ;
#8451=EDGE_CURVE ( 'NONE', #10393, #13274, #2731, .T. ) ;
#8461=CIRCLE ( 'NONE', #4309, 2.500000000000002220 ) ;
#8463=CYLINDRICAL_SURFACE ( 'NONE', #11536, 2.500000000000002220 ) ;
#8470=EDGE_LOOP ( 'NONE', ( #12624, #12127, #12912, #2797 ) ) ;
#8476=CARTESIAN_POINT ( 'NONE',  ( 134.9999999999999432, -56.99999999999997158, -169.9999999999999716 ) ) ;
#8477=ORIENTED_EDGE ( 'NONE', *, *, #3174, .F. ) ;
#8486=VECTOR ( 'NONE', #10699, 1000.000000000000000 ) ;
#8495=VERTEX_POINT ( 'NONE', #9806 ) ;
#8497=ORIENTED_EDGE ( 'NONE', *, *, #6688, .T. ) ;
#8498=DIRECTION ( 'NONE',  ( -0.000000000000000000, -0.000000000000000000, 1.000000000000000000 ) ) ;
#8501=ORIENTED_EDGE ( 'NONE', *, *, #13950, .T. ) ;
#8502=DIRECTION ( 'NONE',  ( -0.000000000000000000, 1.000000000000000000, -0.000000000000000000 ) ) ;
#8508=AXIS2_PLACEMENT_3D ( 'NONE', #10842, #2932, #1832 ) ;
#8511=AXIS2_PLACEMENT_3D ( 'NONE', #6905, #11338, #5819 ) ;
#8512=DIRECTION ( 'NONE',  ( 1.000000000000000000, 0.000000000000000000, 0.000000000000000000 ) ) ;
#8515=EDGE_LOOP ( 'NONE', ( #6627, #12671 ) ) ;
#8517=EDGE_LOOP ( 'NONE', ( #10174, #7608 ) ) ;
#8518=AXIS2_PLACEMENT_3D ( 'NONE', #6388, #14209, #9942 ) ;
#8520=CARTESIAN_POINT ( 'NONE',  ( 305.0000000000000000, -36.99999999999997868, -181.5021515430661054 ) ) ;
#8523=DIRECTION ( 'NONE',  ( 0.000000000000000000, 1.000000000000000000, 0.000000000000000000 ) ) ;
#8524=VECTOR ( 'NONE', #13183, 1000.000000000000000 ) ;
#8534=ORIENTED_EDGE ( 'NONE', *, *, #3563, .T. ) ;
#8536=ADVANCED_FACE ( 'NONE', ( #5718 ), #12006, .F. ) ;
#8544=AXIS2_PLACEMENT_3D ( 'NONE', #12136, #8730, #13151 ) ;
#8546=DIRECTION ( 'NONE',  ( -0.000000000000000000, 1.000000000000000000, -0.000000000000000000 ) ) ;
#8550=VERTEX_POINT ( 'NONE', #10014 ) ;
#8551=DIRECTION ( 'NONE',  ( -1.000000000000000000, 0.000000000000000000, 0.000000000000000000 ) ) ;
#8559=CARTESIAN_POINT ( 'NONE',  ( 299.9999999999999432, -95.00000000000008527, -186.2999999999999829 ) ) ;
#8563=CARTESIAN_POINT ( 'NONE',  ( 140.0000000000000000, -75.00000000000008527, -186.2999999999999829 ) ) ;
#8567=CARTESIAN_POINT ( 'NONE',  ( 303.3333333333333144, -25.00000000000000000, 222.5000000000000853 ) ) ;
#8570=ORIENTED_EDGE ( 'NONE', *, *, #4642, .F. ) ;
#8572=ORIENTED_EDGE ( 'NONE', *, *, #11185, .T. ) ;
#8575=UNCERTAINTY_MEASURE_WITH_UNIT (LENGTH_MEASURE( 1.000000000000000082E-05 ), #1091, 'distance_accuracy_value', 'NONE');
#8576=ORIENTED_EDGE ( 'NONE', *, *, #6222, .F. ) ;
#8578=ORIENTED_EDGE ( 'NONE', *, *, #6768, .F. ) ;
#8579=CARTESIAN_POINT ( 'NONE',  ( 136.6666666666666288, -25.00000000000000000, 222.5000000000000853 ) ) ;
#8580=EDGE_LOOP ( 'NONE', ( #5729, #2845 ) ) ;
#8581=FACE_OUTER_BOUND ( 'NONE', #12215, .T. ) ;
#8584=ADVANCED_FACE ( 'NONE', ( #10076 ), #5734, .F. ) ;
#8587=CARTESIAN_POINT ( 'NONE',  ( 142.6500000000000057, -95.00000000000008527, -169.9999999999999716 ) ) ;
#8592=CARTESIAN_POINT ( 'NONE',  ( -30.00000000000002842, -225.0000000000000000, 169.9999999999999716 ) ) ;
#8594=ORIENTED_EDGE ( 'NONE', *, *, #2946, .T. ) ;
#8597=DIRECTION ( 'NONE',  ( -0.000000000000000000, -0.000000000000000000, 1.000000000000000000 ) ) ;
#8599=CIRCLE ( 'NONE', #11370, 2.500000000000002220 ) ;
#8626=EDGE_LOOP ( 'NONE', ( #1999, #12646 ) ) ;
#8627=AXIS2_PLACEMENT_3D ( 'NONE', #4374, #7548, #8719 ) ;
#8632=ORIENTED_EDGE ( 'NONE', *, *, #11466, .F. ) ;
#8637=CIRCLE ( 'NONE', #4707, 2.649999999999985700 ) ;
#8638=EDGE_LOOP ( 'NONE', ( #9052, #1313, #6802, #5524 ) ) ;
#8640=EDGE_CURVE ( 'NONE', #8550, #11373, #2966, .T. ) ;
#8644=DIRECTION ( 'NONE',  ( 1.000000000000000000, 0.000000000000000000, 0.000000000000000000 ) ) ;
#8649=DIRECTION ( 'NONE',  ( 1.000000000000000000, 0.000000000000000000, 0.000000000000000000 ) ) ;
#8655=DIRECTION ( 'NONE',  ( 0.000000000000000000, 0.000000000000000000, -1.000000000000000000 ) ) ;
#8657=DIRECTION ( 'NONE',  ( 0.000000000000000000, 0.000000000000000000, 1.000000000000000000 ) ) ;
#8658=CARTESIAN_POINT ( 'NONE',  ( 469.9999999999998863, -25.00000000000000000, -190.0000000000000000 ) ) ;
#8666=VECTOR ( 'NONE', #4219, 1000.000000000000000 ) ;
#8667=EDGE_LOOP ( 'NONE', ( #11530, #1951, #4428, #7743 ) ) ;
#8670=FACE_BOUND ( 'NONE', #6148, .T. ) ;
#8671=EDGE_LOOP ( 'NONE', ( #9577, #4697 ) ) ;
#8678=EDGE_CURVE ( 'NONE', #6402, #2854, #5939, .T. ) ;
#8680=DIRECTION ( 'NONE',  ( 1.000000000000000000, 0.000000000000000000, 0.000000000000000000 ) ) ;
#8682=DIRECTION ( 'NONE',  ( 1.000000000000000000, 0.000000000000000000, 0.000000000000000000 ) ) ;
#8688=DIRECTION ( 'NONE',  ( -1.000000000000000000, 0.000000000000000000, 0.000000000000000000 ) ) ;
#8699=ORIENTED_EDGE ( 'NONE', *, *, #5529, .F. ) ;
#8706=PLANE ( 'NONE',  #10170 ) ;
#8711=VECTOR ( 'NONE', #1886, 1000.000000000000000 ) ;
#8718=EDGE_CURVE ( 'NONE', #8809, #12847, #8250, .T. ) ;
#8719=DIRECTION ( 'NONE',  ( 0.000000000000000000, 0.000000000000000000, -1.000000000000000000 ) ) ;
#8728=CARTESIAN_POINT ( 'NONE',  ( 119.9999999999999147, -24.99999999999999289, 19.99999999999998934 ) ) ;
#8730=DIRECTION ( 'NONE',  ( -0.000000000000000000, -0.000000000000000000, 1.000000000000000000 ) ) ;
#8740=FACE_OUTER_BOUND ( 'NONE', #7311, .T. ) ;
#8742=FACE_BOUND ( 'NONE', #5135, .T. ) ;
#8745=VECTOR ( 'NONE', #12070, 1000.000000000000000 ) ;
#8749=LINE ( 'NONE', #3323, #11349 ) ;
#8756=LINE ( 'NONE', #10940, #13214 ) ;
#8758=VECTOR ( 'NONE', #13302, 1000.000000000000000 ) ;
#8759=VERTEX_POINT ( 'NONE', #2605 ) ;
#8765=ORIENTED_EDGE ( 'NONE', *, *, #2122, .F. ) ;
#8766=ADVANCED_FACE ( 'NONE', ( #13831 ), #7026, .F. ) ;
#8771=DIRECTION ( 'NONE',  ( 0.000000000000000000, 1.000000000000000000, 0.000000000000000000 ) ) ;
#8774=EDGE_LOOP ( 'NONE', ( #5235, #6873, #3945, #1369 ) ) ;
#8777=CARTESIAN_POINT ( 'NONE',  ( 0.000000000000000000, 0.000000000000000000, -250.0000000000000000 ) ) ;
#8778=DIRECTION ( 'NONE',  ( -1.000000000000000000, 0.000000000000000000, 0.000000000000000000 ) ) ;
#8783=CARTESIAN_POINT ( 'NONE',  ( 140.0000000000000000, -95.00000000000008527, -190.0000000000000000 ) ) ;
#8787=ORIENTED_EDGE ( 'NONE', *, *, #12071, .T. ) ;
#8788=ADVANCED_FACE ( 'NONE', ( #10357 ), #4130, .F. ) ;
#8795=EDGE_LOOP ( 'NONE', ( #6524, #4487, #8914, #12725 ) ) ;
#8802=ADVANCED_FACE ( 'NONE', ( #833 ), #6294, .F. ) ;
#8809=VERTEX_POINT ( 'NONE', #687 ) ;
#8814=CARTESIAN_POINT ( 'NONE',  ( 142.6500000000000057, -95.00000000000008527, -186.2999999999999829 ) ) ;
#8815=DIRECTION ( 'NONE',  ( -1.000000000000000000, 0.000000000000000000, 0.000000000000000000 ) ) ;
#8816=CIRCLE ( 'NONE', #3496, 2.649999999999985700 ) ;
#8817=ORIENTED_EDGE ( 'NONE', *, *, #7382, .F. ) ;
#8821=AXIS2_PLACEMENT_3D ( 'NONE', #4570, #3617, #8989 ) ;
#8822=DIRECTION ( 'NONE',  ( -0.000000000000000000, -0.000000000000000000, -1.000000000000000000 ) ) ;
#8827=CIRCLE ( 'NONE', #4666, 2.649999999999985700 ) ;
#8828=CARTESIAN_POINT ( 'NONE',  ( 305.0000000000000000, -56.99999999999997158, -169.9999999999999716 ) ) ;
#8838=ORIENTED_EDGE ( 'NONE', *, *, #2375, .T. ) ;
#8842=EDGE_CURVE ( 'NONE', #4959, #7600, #11891, .T. ) ;
#8843=CARTESIAN_POINT ( 'NONE',  ( 236.4999999999999432, -85.00000000000007105, 190.0000000000000000 ) ) ;
#8852=DIRECTION ( 'NONE',  ( -0.000000000000000000, -0.000000000000000000, 1.000000000000000000 ) ) ;
#8857=DIRECTION ( 'NONE',  ( 0.000000000000000000, 0.000000000000000000, 1.000000000000000000 ) ) ;
#8862=ORIENTED_EDGE ( 'NONE', *, *, #800, .F. ) ;
#8865=CYLINDRICAL_SURFACE ( 'NONE', #9786, 2.649999999999985700 ) ;
#8866=VECTOR ( 'NONE', #11221, 1000.000000000000000 ) ;
#8867=VERTEX_POINT ( 'NONE', #7306 ) ;
#8871=FACE_OUTER_BOUND ( 'NONE', #12170, .T. ) ;
#8877=ADVANCED_FACE ( 'NONE', ( #5361 ), #8463, .F. ) ;
#8881=ORIENTED_EDGE ( 'NONE', *, *, #14078, .T. ) ;
#8882=VERTEX_POINT ( 'NONE', #6445 ) ;
#8883=FACE_OUTER_BOUND ( 'NONE', #11268, .T. ) ;
#8886=ORIENTED_EDGE ( 'NONE', *, *, #3049, .F. ) ;
#8890=ORIENTED_EDGE ( 'NONE', *, *, #1154, .F. ) ;
#8902=EDGE_CURVE ( 'NONE', #4007, #10967, #3340, .T. ) ;
#8903=CARTESIAN_POINT ( 'NONE',  ( 303.3333333333333144, -25.00000000000000000, -222.5000000000000853 ) ) ;
#8913=CARTESIAN_POINT ( 'NONE',  ( 219.9999999999999716, -20.00000000000000000, 225.1500000000000625 ) ) ;
#8914=ORIENTED_EDGE ( 'NONE', *, *, #11002, .F. ) ;
#8923=DIRECTION ( 'NONE',  ( 0.000000000000000000, 0.000000000000000000, -1.000000000000000000 ) ) ;
#8929=CARTESIAN_POINT ( 'NONE',  ( 386.6666666666666288, -20.00000000000000000, -222.5000000000000853 ) ) ;
#8930=EDGE_LOOP ( 'NONE', ( #5713, #7181 ) ) ;
#8937=ORIENTED_EDGE ( 'NONE', *, *, #13753, .T. ) ;
#8950=CARTESIAN_POINT ( 'NONE',  ( 470.0000000000000000, -20.00000000000000000, 250.0000000000000000 ) ) ;
#8952=CIRCLE ( 'NONE', #3856, 2.649999999999985700 ) ;
#8963=CARTESIAN_POINT ( 'NONE',  ( 302.5000000000000000, -36.99999999999997868, -180.0000000000000000 ) ) ;
#8968=AXIS2_PLACEMENT_3D ( 'NONE', #481, #8046, #1509 ) ;
#8976=ADVANCED_FACE ( 'NONE', ( #8871 ), #2474, .F. ) ;
#8977=AXIS2_PLACEMENT_3D ( 'NONE', #6742, #4569, #10219 ) ;
#8979=VECTOR ( 'NONE', #11538, 1000.000000000000000 ) ;
#8985=FACE_OUTER_BOUND ( 'NONE', #9346, .T. ) ;
#8986=CARTESIAN_POINT ( 'NONE',  ( 303.3333333333333144, -20.00000000000000000, 219.8500000000001080 ) ) ;
#8989=DIRECTION ( 'NONE',  ( -1.000000000000000000, 0.000000000000000000, 0.000000000000000000 ) ) ;
#8991=LINE ( 'NONE', #2106, #13810 ) ;
#8997=CARTESIAN_POINT ( 'NONE',  ( 305.0000000000000000, -56.99999999999997158, -169.9999999999999716 ) ) ;
#8999=ORIENTED_EDGE ( 'NONE', *, *, #7206, .F. ) ;
#9008=DIRECTION ( 'NONE',  ( -0.000000000000000000, -0.000000000000000000, -1.000000000000000000 ) ) ;
#9015=VERTEX_POINT ( 'NONE', #12522 ) ;
#9018=EDGE_CURVE ( 'NONE', #12143, #1416, #595, .T. ) ;
#9026=EDGE_CURVE ( 'NONE', #11223, #12345, #9898, .T. ) ;
#9027=LINE ( 'NONE', #7065, #2544 ) ;
#9028=DIRECTION ( 'NONE',  ( 0.000000000000000000, 0.000000000000000000, -1.000000000000000000 ) ) ;
#9036=CARTESIAN_POINT ( 'NONE',  ( 305.0000000000000000, -56.99999999999997158, -180.0000000000000000 ) ) ;
#9042=CIRCLE ( 'NONE', #2087, 2.500000000000002220 ) ;
#9046=DIRECTION ( 'NONE',  ( 0.000000000000000000, -1.000000000000000000, 0.000000000000000000 ) ) ;
#9048=DIRECTION ( 'NONE',  ( -0.000000000000000000, -0.000000000000000000, 1.000000000000000000 ) ) ;
#9050=VECTOR ( 'NONE', #897, 1000.000000000000000 ) ;
#9051=EDGE_LOOP ( 'NONE', ( #4157, #4736, #4415, #8890 ) ) ;
#9052=ORIENTED_EDGE ( 'NONE', *, *, #1610, .F. ) ;
#9060=DIRECTION ( 'NONE',  ( -1.000000000000000000, 0.000000000000000000, 0.000000000000000000 ) ) ;
#9065=ORIENTED_EDGE ( 'NONE', *, *, #13449, .T. ) ;
#9066=ORIENTED_EDGE ( 'NONE', *, *, #3817, .T. ) ;
#9068=ORIENTED_EDGE ( 'NONE', *, *, #7615, .F. ) ;
#9069=FACE_OUTER_BOUND ( 'NONE', #2618, .T. ) ;
#9070=ADVANCED_FACE ( 'NONE', ( #7010 ), #4914, .F. ) ;
#9075=CARTESIAN_POINT ( 'NONE',  ( 305.0000000000000000, -56.99999999999997158, -169.9999999999999716 ) ) ;
#9081=CARTESIAN_POINT ( 'NONE',  ( 303.3333333333333144, -20.00000000000000000, 222.5000000000000853 ) ) ;
#9086=DIRECTION ( 'NONE',  ( 0.000000000000000000, 0.000000000000000000, -1.000000000000000000 ) ) ;
#9097=ORIENTED_EDGE ( 'NONE', *, *, #2035, .F. ) ;
#9106=EDGE_CURVE ( 'NONE', #7861, #13795, #1479, .T. ) ;
#9107=VERTEX_POINT ( 'NONE', #375 ) ;
#9109=CYLINDRICAL_SURFACE ( 'NONE', #2344, 2.649999999999985700 ) ;
#9111=CARTESIAN_POINT ( 'NONE',  ( 145.5000000000000284, -95.00000000000008527, -190.0000000000000000 ) ) ;
#9120=VERTEX_POINT ( 'NONE', #5064 ) ;
#9126=FACE_BOUND ( 'NONE', #14100, .T. ) ;
#9129=DIRECTION ( 'NONE',  ( -0.000000000000000000, -0.000000000000000000, 1.000000000000000000 ) ) ;
#9134=ORIENTED_EDGE ( 'NONE', *, *, #8842, .F. ) ;
#9136=VERTEX_POINT ( 'NONE', #4984 ) ;
#9137=CARTESIAN_POINT ( 'NONE',  ( 119.9999999999999147, -20.00000000000000000, -169.9999999999999716 ) ) ;
#9138=ADVANCED_FACE ( 'NONE', ( #12591 ), #2654, .F. ) ;
#9142=DIRECTION ( 'NONE',  ( 1.000000000000000000, 0.000000000000000000, -0.000000000000000000 ) ) ;
#9145=DIRECTION ( 'NONE',  ( -1.000000000000000000, 0.000000000000000000, 0.000000000000000000 ) ) ;
#9148=FACE_OUTER_BOUND ( 'NONE', #398, .T. ) ;
#9151=ADVANCED_FACE ( 'NONE', ( #8450 ), #887, .F. ) ;
#9157=EDGE_LOOP ( 'NONE', ( #8817, #3473 ) ) ;
#9159=CARTESIAN_POINT ( 'NONE',  ( 469.9999999999998863, -225.0000000000000000, 190.0000000000000000 ) ) ;
#9168=DIRECTION ( 'NONE',  ( -0.000000000000000000, -0.000000000000000000, -1.000000000000000000 ) ) ;
#9170=ORIENTED_EDGE ( 'NONE', *, *, #13243, .F. ) ;
#9171=AXIS2_PLACEMENT_3D ( 'NONE', #12114, #6671, #1134 ) ;
#9177=ADVANCED_FACE ( 'NONE', ( #746 ), #9995, .F. ) ;
#9178=EDGE_LOOP ( 'NONE', ( #1072, #3364, #12555, #3710 ) ) ;
#9179=AXIS2_PLACEMENT_3D ( 'NONE', #12030, #12969, #4128 ) ;
#9186=DIRECTION ( 'NONE',  ( -1.000000000000000000, 0.000000000000000000, 0.000000000000000000 ) ) ;
#9187=CIRCLE ( 'NONE', #4104, 2.500000000000002220 ) ;
#9193=AXIS2_PLACEMENT_3D ( 'NONE', #4303, #14299, #2689 ) ;
#9195=ORIENTED_EDGE ( 'NONE', *, *, #9345, .T. ) ;
#9201=CARTESIAN_POINT ( 'NONE',  ( 219.9999999999999716, -85.00000000000007105, 169.9999999999999716 ) ) ;
#9204=CARTESIAN_POINT ( 'NONE',  ( 307.5000000000000000, -56.99999999999997158, -169.9999999999999716 ) ) ;
#9205=DIRECTION ( 'NONE',  ( -0.000000000000000000, 1.000000000000000000, -0.000000000000000000 ) ) ;
#9214=CARTESIAN_POINT ( 'NONE',  ( 219.9999999999999716, -25.00000000000000000, 222.5000000000000853 ) ) ;
#9217=DIRECTION ( 'NONE',  ( 0.000000000000000000, 0.000000000000000000, 1.000000000000000000 ) ) ;
#9218=ORIENTED_EDGE ( 'NONE', *, *, #5882, .F. ) ;
#9219=CARTESIAN_POINT ( 'NONE',  ( 219.9999999999999716, -85.00000000000007105, -250.0009999999999764 ) ) ;
#9229=CARTESIAN_POINT ( 'NONE',  ( 297.3499999999999659, -75.00000000000008527, -186.2999999999999829 ) ) ;
#9235=FACE_BOUND ( 'NONE', #12023, .T. ) ;
#9240=ADVANCED_FACE ( 'NONE', ( #11872 ), #13090, .F. ) ;
#9241=EDGE_CURVE ( 'NONE', #2854, #1558, #6356, .T. ) ;
#9243=DIRECTION ( 'NONE',  ( -1.000000000000000000, 0.000000000000000000, 0.000000000000000000 ) ) ;
#9246=VECTOR ( 'NONE', #7889, 1000.000000000000000 ) ;
#9268=DIRECTION ( 'NONE',  ( -0.000000000000000000, -0.000000000000000000, 1.000000000000000000 ) ) ;
#9271=ORIENTED_EDGE ( 'NONE', *, *, #13042, .F. ) ;
#9279=DIRECTION ( 'NONE',  ( 0.000000000000000000, 1.000000000000000000, 0.000000000000000000 ) ) ;
#9282=FACE_OUTER_BOUND ( 'NONE', #1487, .T. ) ;
#9304=CARTESIAN_POINT ( 'NONE',  ( 140.0000000000000000, -95.00000000000008527, 190.0000000000000000 ) ) ;
#9309=DIRECTION ( 'NONE',  ( 0.000000000000000000, 0.000000000000000000, 1.000000000000000000 ) ) ;
#9314=EDGE_CURVE ( 'NONE', #1382, #4602, #3454, .T. ) ;
#9327=( NAMED_UNIT ( * ) SI_UNIT ( $, .STERADIAN. ) SOLID_ANGLE_UNIT ( ) );
#9328=ORIENTED_EDGE ( 'NONE', *, *, #7382, .T. ) ;
#9334=DIRECTION ( 'NONE',  ( 0.000000000000000000, 0.000000000000000000, -1.000000000000000000 ) ) ;
#9336=CYLINDRICAL_SURFACE ( 'NONE', #13669, 2.500000000000002220 ) ;
#9337=CARTESIAN_POINT ( 'NONE',  ( 303.3333333333333144, -20.00000000000000000, 222.5000000000000853 ) ) ;
#9343=AXIS2_PLACEMENT_3D ( 'NONE', #6525, #8771, #7528 ) ;
#9345=EDGE_CURVE ( 'NONE', #7698, #10393, #6711, .T. ) ;
#9346=EDGE_LOOP ( 'NONE', ( #4226, #13342, #96, #736 ) ) ;
#9347=CARTESIAN_POINT ( 'NONE',  ( 140.0000000000000000, -75.00000000000008527, 190.0000000000000000 ) ) ;
#9354=DIRECTION ( 'NONE',  ( -0.000000000000000000, 1.000000000000000000, -0.000000000000000000 ) ) ;
#9360=DIRECTION ( 'NONE',  ( 0.000000000000000000, 0.000000000000000000, 1.000000000000000000 ) ) ;
#9363=DIRECTION ( 'NONE',  ( 1.000000000000000000, 0.000000000000000000, 0.000000000000000000 ) ) ;
#9364=ORIENTED_EDGE ( 'NONE', *, *, #8416, .F. ) ;
#9375=LINE ( 'NONE', #12628, #5045 ) ;
#9378=VECTOR ( 'NONE', #12126, 1000.000000000000000 ) ;
#9382=CARTESIAN_POINT ( 'NONE',  ( 145.5000000000000284, -95.00000000000008527, 190.0000000000000000 ) ) ;
#9384=DIRECTION ( 'NONE',  ( -0.000000000000000000, -0.000000000000000000, 1.000000000000000000 ) ) ;
#9387=AXIS2_PLACEMENT_3D ( 'NONE', #8997, #3493, #7896 ) ;
#9390=CARTESIAN_POINT ( 'NONE',  ( 299.9999999999999432, -95.00000000000008527, -190.0000000000000000 ) ) ;
#9393=EDGE_CURVE ( 'NONE', #6403, #10296, #1638, .T. ) ;
#9396=ORIENTED_EDGE ( 'NONE', *, *, #12971, .F. ) ;
#9403=DIRECTION ( 'NONE',  ( -0.000000000000000000, -0.000000000000000000, -1.000000000000000000 ) ) ;
#9411=CARTESIAN_POINT ( 'NONE',  ( 137.3500000000000227, -95.00000000000008527, 186.2999999999999829 ) ) ;
#9413=VERTEX_POINT ( 'NONE', #11076 ) ;
#9415=EDGE_CURVE ( 'NONE', #13552, #6403, #76, .T. ) ;
#9418=DIRECTION ( 'NONE',  ( 0.000000000000000000, 0.000000000000000000, 1.000000000000000000 ) ) ;
#9420=DIRECTION ( 'NONE',  ( -1.000000000000000000, 0.000000000000000000, 0.000000000000000000 ) ) ;
#9428=AXIS2_PLACEMENT_3D ( 'NONE', #11423, #1466, #5902 ) ;
#9429=ORIENTED_EDGE ( 'NONE', *, *, #10092, .F. ) ;
#9438=ORIENTED_EDGE ( 'NONE', *, *, #11811, .T. ) ;
#9439=LINE ( 'NONE', #10524, #14035 ) ;
#9443=EDGE_CURVE ( 'NONE', #10838, #1381, #936, .T. ) ;
#9448=DIRECTION ( 'NONE',  ( -0.000000000000000000, -0.000000000000000000, -1.000000000000000000 ) ) ;
#9450=CIRCLE ( 'NONE', #14064, 2.649999999999985700 ) ;
#9452=ORIENTED_EDGE ( 'NONE', *, *, #2851, .T. ) ;
#9454=AXIS2_PLACEMENT_3D ( 'NONE', #8563, #4068, #8778 ) ;
#9463=CARTESIAN_POINT ( 'NONE',  ( 137.3500000000000227, -95.00000000000008527, -186.2999999999999829 ) ) ;
#9464=DIRECTION ( 'NONE',  ( -0.000000000000000000, -0.000000000000000000, 1.000000000000000000 ) ) ;
#9467=ORIENTED_EDGE ( 'NONE', *, *, #12977, .T. ) ;
#9474=VERTEX_POINT ( 'NONE', #13512 ) ;
#9481=ORIENTED_EDGE ( 'NONE', *, *, #704, .F. ) ;
#9482=AXIS2_PLACEMENT_3D ( 'NONE', #8162, #3814, #13603 ) ;
#9483=CARTESIAN_POINT ( 'NONE',  ( 299.9999999999999432, -75.00000000000008527, 186.2999999999999829 ) ) ;
#9485=CARTESIAN_POINT ( 'NONE',  ( 303.3333333333333144, -25.00000000000000000, -219.8500000000001080 ) ) ;
#9491=DIRECTION ( 'NONE',  ( -0.000000000000000000, -1.000000000000000000, -0.000000000000000000 ) ) ;
#9498=AXIS2_PLACEMENT_3D ( 'NONE', #9081, #8053, #1454 ) ;
#9507=CIRCLE ( 'NONE', #3264, 2.649999999999985700 ) ;
#9512=EDGE_CURVE ( 'NONE', #9107, #10453, #11390, .T. ) ;
#9518=DIRECTION ( 'NONE',  ( -0.000000000000000000, -0.000000000000000000, 1.000000000000000000 ) ) ;
#9521=VECTOR ( 'NONE', #6382, 1000.000000000000000 ) ;
#9527=ORIENTED_EDGE ( 'NONE', *, *, #5626, .F. ) ;
#9531=CARTESIAN_POINT ( 'NONE',  ( 219.9999999999999716, -25.00000000000000000, 222.5000000000000853 ) ) ;
#9532=ORIENTED_EDGE ( 'NONE', *, *, #7087, .F. ) ;
#9537=FACE_BOUND ( 'NONE', #7943, .T. ) ;
#9539=FACE_OUTER_BOUND ( 'NONE', #6458, .T. ) ;
#9541=( NAMED_UNIT ( * ) SI_UNIT ( $, .STERADIAN. ) SOLID_ANGLE_UNIT ( ) );
#9544=ORIENTED_EDGE ( 'NONE', *, *, #4088, .T. ) ;
#9548=FACE_BOUND ( 'NONE', #11231, .T. ) ;
#9550=VECTOR ( 'NONE', #10223, 1000.000000000000000 ) ;
#9554=CARTESIAN_POINT ( 'NONE',  ( 134.5000000000000000, -75.00000000000008527, 190.0000000000000000 ) ) ;
#9556=MECHANICAL_DESIGN_GEOMETRIC_PRESENTATION_REPRESENTATION('',(#7463),#2847);
#9557=LINE ( 'NONE', #2958, #1851 ) ;
#9558=AXIS2_PLACEMENT_3D ( 'NONE', #13627, #2469, #3701 ) ;
#9560=ORIENTED_EDGE ( 'NONE', *, *, #11029, .T. ) ;
#9563=LINE ( 'NONE', #1785, #8114 ) ;
#9576=CARTESIAN_POINT ( 'NONE',  ( 53.33333333333330017, -25.00000000000000000, -222.5000000000000853 ) ) ;
#9577=ORIENTED_EDGE ( 'NONE', *, *, #1827, .T. ) ;
#9579=CARTESIAN_POINT ( 'NONE',  ( 299.9999999999999432, -75.00000000000008527, 169.9999999999999716 ) ) ;
#9581=CARTESIAN_POINT ( 'NONE',  ( 137.4999999999999432, -56.99999999999997158, -180.0000000000000000 ) ) ;
#9584=LINE ( 'NONE', #11607, #2734 ) ;
#9591=LINE ( 'NONE', #7409, #4182 ) ;
#9594=ORIENTED_EDGE ( 'NONE', *, *, #5946, .T. ) ;
#9595=ORIENTED_EDGE ( 'NONE', *, *, #13449, .F. ) ;
#9596=EDGE_CURVE ( 'NONE', #11916, #6940, #5904, .T. ) ;
#9606=DIRECTION ( 'NONE',  ( -0.000000000000000000, 1.000000000000000000, -0.000000000000000000 ) ) ;
#9607=CARTESIAN_POINT ( 'NONE',  ( -30.00000000000002842, -225.0000000000000000, 169.9999999999999716 ) ) ;
#9608=EDGE_CURVE ( 'NONE', #8094, #5470, #13940, .T. ) ;
#9609=ADVANCED_FACE ( 'NONE', ( #9539 ), #13948, .F. ) ;
#9614=AXIS2_PLACEMENT_3D ( 'NONE', #982, #4423, #5432 ) ;
#9616=ORIENTED_EDGE ( 'NONE', *, *, #5803, .F. ) ;
#9618=DIRECTION ( 'NONE',  ( -0.000000000000000000, -0.000000000000000000, 1.000000000000000000 ) ) ;
#9625=CARTESIAN_POINT ( 'NONE',  ( -30.00000000000002842, -25.00000000000000000, 169.9999999999999716 ) ) ;
#9627=ORIENTED_EDGE ( 'NONE', *, *, #5593, .F. ) ;
#9634=CARTESIAN_POINT ( 'NONE',  ( 140.0000000000000000, -95.00000000000008527, -190.0000000000000000 ) ) ;
#9645=VERTEX_POINT ( 'NONE', #6603 ) ;
#9648=CARTESIAN_POINT ( 'NONE',  ( 294.4999999999999432, -95.00000000000008527, 190.0000000000000000 ) ) ;
#9652=VERTEX_POINT ( 'NONE', #6263 ) ;
#9655=EDGE_LOOP ( 'NONE', ( #11778, #6749 ) ) ;
#9666=ORIENTED_EDGE ( 'NONE', *, *, #2431, .T. ) ;
#9672=ORIENTED_EDGE ( 'NONE', *, *, #6410, .F. ) ;
#9676=VERTEX_POINT ( 'NONE', #995 ) ;
#9677=CARTESIAN_POINT ( 'NONE',  ( 219.9999999999999716, -25.00000000000000000, 219.8500000000001080 ) ) ;
#9678=CIRCLE ( 'NONE', #9193, 5.500000000000005329 ) ;
#9680=VECTOR ( 'NONE', #7274, 1000.000000000000000 ) ;
#9685=VECTOR ( 'NONE', #13501, 1000.000000000000000 ) ;
#9691=ORIENTED_EDGE ( 'NONE', *, *, #11575, .F. ) ;
#9694=ORIENTED_EDGE ( 'NONE', *, *, #6222, .T. ) ;
#9698=FACE_BOUND ( 'NONE', #1348, .T. ) ;
#9699=ORIENTED_EDGE ( 'NONE', *, *, #7150, .F. ) ;
#9700=EDGE_CURVE ( 'NONE', #10145, #2569, #9780, .T. ) ;
#9702=DIRECTION ( 'NONE',  ( 0.000000000000000000, 0.000000000000000000, -1.000000000000000000 ) ) ;
#9706=ORIENTED_EDGE ( 'NONE', *, *, #6997, .T. ) ;
#9726=ORIENTED_EDGE ( 'NONE', *, *, #3318, .T. ) ;
#9732=VERTEX_POINT ( 'NONE', #4435 ) ;
#9735=EDGE_CURVE ( 'NONE', #5871, #11569, #13251, .T. ) ;
#9739=VERTEX_POINT ( 'NONE', #5046 ) ;
#9740=VERTEX_POINT ( 'NONE', #6122 ) ;
#9742=VERTEX_POINT ( 'NONE', #9463 ) ;
#9744=CARTESIAN_POINT ( 'NONE',  ( 299.9999999999999432, -95.00000000000008527, 190.0000000000000000 ) ) ;
#9757=ORIENTED_EDGE ( 'NONE', *, *, #11621, .T. ) ;
#9759=EDGE_LOOP ( 'NONE', ( #9170, #364, #3428, #5373 ) ) ;
#9776=CARTESIAN_POINT ( 'NONE',  ( 137.4999999999999432, -36.99999999999997868, -180.0000000000000000 ) ) ;
#9780=CIRCLE ( 'NONE', #2134, 5.500000000000005329 ) ;
#9786=AXIS2_PLACEMENT_3D ( 'NONE', #7762, #4299, #10833 ) ;
#9788=EDGE_CURVE ( 'NONE', #5508, #328, #1281, .T. ) ;
#9789=CARTESIAN_POINT ( 'NONE',  ( 140.0000000000000000, -95.00000000000008527, 190.0000000000000000 ) ) ;
#9790=EDGE_CURVE ( 'NONE', #9959, #2372, #2535, .T. ) ;
#9798=CARTESIAN_POINT ( 'NONE',  ( -30.00000000000002842, -225.0000000000000000, 190.0000000000000000 ) ) ;
#9800=ORIENTED_EDGE ( 'NONE', *, *, #7894, .T. ) ;
#9804=AXIS2_PLACEMENT_3D ( 'NONE', #8273, #13926, #2769 ) ;
#9806=CARTESIAN_POINT ( 'NONE',  ( 302.6499999999999204, -75.00000000000008527, -169.9999999999999716 ) ) ;
#9807=DIRECTION ( 'NONE',  ( 0.000000000000000000, 1.000000000000000000, 0.000000000000000000 ) ) ;
#9812=ORIENTED_EDGE ( 'NONE', *, *, #3673, .T. ) ;
#9814=DIRECTION ( 'NONE',  ( 1.000000000000000000, 0.000000000000000000, 0.000000000000000000 ) ) ;
#9815=ORIENTED_EDGE ( 'NONE', *, *, #1803, .T. ) ;
#9822=DIRECTION ( 'NONE',  ( -0.000000000000000000, 0.000000000000000000, 1.000000000000000000 ) ) ;
#9823=DIRECTION ( 'NONE',  ( 0.000000000000000000, 1.000000000000000000, 0.000000000000000000 ) ) ;
#9827=DIRECTION ( 'NONE',  ( 1.000000000000000000, 0.000000000000000000, 0.000000000000000000 ) ) ;
#9830=CARTESIAN_POINT ( 'NONE',  ( 53.33333333333330017, -20.00000000000000000, 222.5000000000000853 ) ) ;
#9833=DIRECTION ( 'NONE',  ( 1.000000000000000000, 0.000000000000000000, -0.000000000000000000 ) ) ;
#9834=FACE_BOUND ( 'NONE', #2082, .T. ) ;
#9837=CARTESIAN_POINT ( 'NONE',  ( 297.3499999999999659, -95.00000000000008527, -190.0000000000000000 ) ) ;
#9839=DIRECTION ( 'NONE',  ( 1.000000000000000000, 0.000000000000000000, 0.000000000000000000 ) ) ;
#9842=ORIENTED_EDGE ( 'NONE', *, *, #504, .F. ) ;
#9843=EDGE_LOOP ( 'NONE', ( #4019, #11712, #265, #12536 ) ) ;
#9844=CARTESIAN_POINT ( 'NONE',  ( -30.00000000000002842, -20.00000000000000000, -250.0000000000000000 ) ) ;
#9846=CARTESIAN_POINT ( 'NONE',  ( 119.9999999999999147, -20.00000000000000000, 169.9999999999999716 ) ) ;
#9856=DIRECTION ( 'NONE',  ( 1.000000000000000000, 0.000000000000000000, 0.000000000000000000 ) ) ;
#9859=DIRECTION ( 'NONE',  ( -1.000000000000000000, 0.000000000000000000, 0.000000000000000000 ) ) ;
#9860=ADVANCED_FACE ( 'NONE', ( #12327 ), #13538, .F. ) ;
#9865=EDGE_CURVE ( 'NONE', #1020, #12884, #13406, .T. ) ;
#9870=DIRECTION ( 'NONE',  ( -0.000000000000000000, 0.000000000000000000, 1.000000000000000000 ) ) ;
#9871=CARTESIAN_POINT ( 'NONE',  ( 305.0000000000000000, -36.99999999999997868, -180.0000000000000000 ) ) ;
#9872=FACE_OUTER_BOUND ( 'NONE', #6965, .T. ) ;
#9873=CARTESIAN_POINT ( 'NONE',  ( 299.9999999999999432, -95.00000000000008527, 186.2999999999999829 ) ) ;
#9877=ORIENTED_EDGE ( 'NONE', *, *, #12521, .F. ) ;
#9880=EDGE_LOOP ( 'NONE', ( #4673, #7981 ) ) ;
#9887=CARTESIAN_POINT ( 'NONE',  ( 142.6500000000000057, -95.00000000000008527, 186.2999999999999829 ) ) ;
#9895=CARTESIAN_POINT ( 'NONE',  ( 137.3500000000000227, -75.00000000000008527, 186.2999999999999829 ) ) ;
#9898=CIRCLE ( 'NONE', #10115, 2.649999999999985700 ) ;
#9899=ORIENTED_EDGE ( 'NONE', *, *, #1597, .T. ) ;
#9900=AXIS2_PLACEMENT_3D ( 'NONE', #6171, #2629, #2843 ) ;
#9909=ORIENTED_EDGE ( 'NONE', *, *, #3196, .T. ) ;
#9910=CIRCLE ( 'NONE', #9454, 5.500000000000005329 ) ;
#9911=DIRECTION ( 'NONE',  ( 0.000000000000000000, 0.000000000000000000, 1.000000000000000000 ) ) ;
#9912=CIRCLE ( 'NONE', #5726, 5.500000000000005329 ) ;
#9917=ORIENTED_EDGE ( 'NONE', *, *, #5694, .F. ) ;
#9918=FACE_OUTER_BOUND ( 'NONE', #10891, .T. ) ;
#9921=VECTOR ( 'NONE', #3521, 1000.000000000000000 ) ;
#9925=CYLINDRICAL_SURFACE ( 'NONE', #5769, 2.649999999999985700 ) ;
#9929=ORIENTED_EDGE ( 'NONE', *, *, #12338, .T. ) ;
#9934=FACE_OUTER_BOUND ( 'NONE', #6514, .T. ) ;
#9936=EDGE_CURVE ( 'NONE', #8189, #7589, #107, .T. ) ;
#9942=DIRECTION ( 'NONE',  ( 0.000000000000000000, 0.000000000000000000, -1.000000000000000000 ) ) ;
#9947=FACE_OUTER_BOUND ( 'NONE', #2706, .T. ) ;
#9957=EDGE_CURVE ( 'NONE', #3293, #3594, #3833, .T. ) ;
#9959=VERTEX_POINT ( 'NONE', #11451 ) ;
#9961=ORIENTED_EDGE ( 'NONE', *, *, #6248, .F. ) ;
#9962=VECTOR ( 'NONE', #1109, 1000.000000000000000 ) ;
#9968=EDGE_CURVE ( 'NONE', #8495, #10689, #10511, .T. ) ;
#9972=EDGE_CURVE ( 'NONE', #1006, #8809, #1568, .T. ) ;
#9978=EDGE_LOOP ( 'NONE', ( #6020, #13268, #8570, #4080 ) ) ;
#9981=LINE ( 'NONE', #1183, #8758 ) ;
#9982=ORIENTED_EDGE ( 'NONE', *, *, #6482, .T. ) ;
#9988=CYLINDRICAL_SURFACE ( 'NONE', #2561, 2.500000000000002220 ) ;
#9995=CONICAL_SURFACE ( 'NONE', #10458, 2.500000000000002220, 1.029744260000002631 ) ;
#10002=ORIENTED_EDGE ( 'NONE', *, *, #1882, .F. ) ;
#10010=EDGE_LOOP ( 'NONE', ( #7017, #13526, #11985, #9666 ) ) ;
#10013=LINE ( 'NONE', #8986, #14303 ) ;
#10014=CARTESIAN_POINT ( 'NONE',  ( 209.9999999999999716, -85.00000000000007105, 169.9999999999999716 ) ) ;
#10030=AXIS2_PLACEMENT_3D ( 'NONE', #1, #2352, #948 ) ;
#10041=PLANE ( 'NONE',  #12676 ) ;
#10042=AXIS2_PLACEMENT_3D ( 'NONE', #7251, #3918, #7172 ) ;
#10043=VERTEX_POINT ( 'NONE', #390 ) ;
#10044=EDGE_LOOP ( 'NONE', ( #10740, #10716, #3689, #7938 ) ) ;
#10046=ORIENTED_EDGE ( 'NONE', *, *, #13299, .F. ) ;
#10047=CARTESIAN_POINT ( 'NONE',  ( 136.6666666666666288, -20.00000000000000000, -222.5000000000000853 ) ) ;
#10063=DIRECTION ( 'NONE',  ( -0.000000000000000000, -0.000000000000000000, 1.000000000000000000 ) ) ;
#10067=CARTESIAN_POINT ( 'NONE',  ( 219.9999999999999716, -25.00000000000000000, -219.8500000000001080 ) ) ;
#10072=CYLINDRICAL_SURFACE ( 'NONE', #6160, 5.500000000000005329 ) ;
#10076=FACE_OUTER_BOUND ( 'NONE', #5951, .T. ) ;
#10077=CARTESIAN_POINT ( 'NONE',  ( 303.3333333333333144, -20.00000000000000000, 219.8500000000001080 ) ) ;
#10079=DIRECTION ( 'NONE',  ( -0.000000000000000000, 0.000000000000000000, 1.000000000000000000 ) ) ;
#10082=ORIENTED_EDGE ( 'NONE', *, *, #11731, .F. ) ;
#10092=EDGE_CURVE ( 'NONE', #634, #2924, #10268, .T. ) ;
#10094=FACE_OUTER_BOUND ( 'NONE', #6906, .T. ) ;
#10100=CARTESIAN_POINT ( 'NONE',  ( 137.4999999999999432, -56.99999999999997158, -169.9999999999999716 ) ) ;
#10101=ORIENTED_EDGE ( 'NONE', *, *, #7615, .T. ) ;
#10108=CARTESIAN_POINT ( 'NONE',  ( -30.00000000000002842, -25.00000000000000000, 250.0000000000000000 ) ) ;
#10109=AXIS2_PLACEMENT_3D ( 'NONE', #10856, #5058, #11792 ) ;
#10114=CARTESIAN_POINT ( 'NONE',  ( 470.0000000000000000, -25.00000000000000000, -169.9999999999999716 ) ) ;
#10115=AXIS2_PLACEMENT_3D ( 'NONE', #11655, #10418, #12452 ) ;
#10128=AXIS2_PLACEMENT_3D ( 'NONE', #3781, #13553, #9142 ) ;
#10133=AXIS2_PLACEMENT_3D ( 'NONE', #12846, #6176, #3857 ) ;
#10138=EDGE_LOOP ( 'NONE', ( #11984, #13055, #2891, #3878 ) ) ;
#10140=CARTESIAN_POINT ( 'NONE',  ( 305.4999999999999432, -75.00000000000008527, 190.0000000000000000 ) ) ;
#10145=VERTEX_POINT ( 'NONE', #12307 ) ;
#10146=CARTESIAN_POINT ( 'NONE',  ( 236.4999999999999432, -85.00000000000007105, 190.0000000000000000 ) ) ;
#10150=DIRECTION ( 'NONE',  ( -0.000000000000000000, 1.000000000000000000, -0.000000000000000000 ) ) ;
#10151=CARTESIAN_POINT ( 'NONE',  ( 140.0000000000000000, -95.00000000000008527, 190.0000000000000000 ) ) ;
#10152=DIRECTION ( 'NONE',  ( 0.000000000000000000, 0.000000000000000000, -1.000000000000000000 ) ) ;
#10163=CONICAL_SURFACE ( 'NONE', #11328, 2.500000000000002220, 1.029744260000002631 ) ;
#10164=LINE ( 'NONE', #124, #4766 ) ;
#10170=AXIS2_PLACEMENT_3D ( 'NONE', #13334, #9870, #10968 ) ;
#10173=FACE_BOUND ( 'NONE', #13994, .T. ) ;
#10174=ORIENTED_EDGE ( 'NONE', *, *, #872, .F. ) ;
#10196=CARTESIAN_POINT ( 'NONE',  ( 219.9999999999999716, -20.00000000000000000, 219.8500000000001080 ) ) ;
#10198=EDGE_LOOP ( 'NONE', ( #8117, #12714 ) ) ;
#10212=CIRCLE ( 'NONE', #3285, 2.649999999999985700 ) ;
#10217=ADVANCED_FACE ( 'NONE', ( #1847 ), #1767, .F. ) ;
#10219=DIRECTION ( 'NONE',  ( 1.000000000000000000, 0.000000000000000000, 0.000000000000000000 ) ) ;
#10221=CIRCLE ( 'NONE', #3969, 2.500000000000002220 ) ;
#10223=DIRECTION ( 'NONE',  ( -0.8571673013836870192, 1.049727191973306873E-16, 0.5150380737757234151 ) ) ;
#10234=DIRECTION ( 'NONE',  ( -0.000000000000000000, -1.000000000000000000, -0.000000000000000000 ) ) ;
#10236=CARTESIAN_POINT ( 'NONE',  ( 294.4999999999999432, -95.00000000000008527, 186.2999999999999829 ) ) ;
#10237=DIRECTION ( 'NONE',  ( -1.000000000000000000, 0.000000000000000000, 0.000000000000000000 ) ) ;
#10248=ORIENTED_EDGE ( 'NONE', *, *, #11946, .T. ) ;
#10250=CARTESIAN_POINT ( 'NONE',  ( 303.3333333333333144, -20.00000000000000000, -222.5000000000000853 ) ) ;
#10254=ORIENTED_EDGE ( 'NONE', *, *, #8718, .T. ) ;
#10256=ORIENTED_EDGE ( 'NONE', *, *, #2241, .F. ) ;
#10259=VECTOR ( 'NONE', #8523, 1000.000000000000000 ) ;
#10260=DIRECTION ( 'NONE',  ( -0.000000000000000000, 1.000000000000000000, -0.000000000000000000 ) ) ;
#10261=FACE_OUTER_BOUND ( 'NONE', #6305, .T. ) ;
#10262=CARTESIAN_POINT ( 'NONE',  ( 145.5000000000000284, -75.00000000000008527, -190.0000000000000000 ) ) ;
#10263=CARTESIAN_POINT ( 'NONE',  ( 219.9999999999999716, -20.00000000000000000, 222.5000000000000853 ) ) ;
#10268=LINE ( 'NONE', #4619, #8866 ) ;
#10272=CARTESIAN_POINT ( 'NONE',  ( 305.4999999999999432, -95.00000000000008527, 190.0000000000000000 ) ) ;
#10291=EDGE_LOOP ( 'NONE', ( #3629, #4893, #11994, #12614 ) ) ;
#10296=VERTEX_POINT ( 'NONE', #670 ) ;
#10297=CARTESIAN_POINT ( 'NONE',  ( -30.00000000000002842, -20.00000000000000000, 250.0000000000000000 ) ) ;
#10299=PLANE ( 'NONE',  #10128 ) ;
#10300=VERTEX_POINT ( 'NONE', #2651 ) ;
#10303=LINE ( 'NONE', #3709, #144 ) ;
#10311=EDGE_LOOP ( 'NONE', ( #6547, #3157 ) ) ;
#10315=VERTEX_POINT ( 'NONE', #8376 ) ;
#10317=ORIENTED_EDGE ( 'NONE', *, *, #10554, .F. ) ;
#10319=EDGE_LOOP ( 'NONE', ( #10980, #8881 ) ) ;
#10322=AXIS2_PLACEMENT_3D ( 'NONE', #7630, #3296, #10909 ) ;
#10323=DIRECTION ( 'NONE',  ( 0.000000000000000000, 0.000000000000000000, 1.000000000000000000 ) ) ;
#10326=CARTESIAN_POINT ( 'NONE',  ( -30.00000000000002842, -25.00000000000000000, -250.0000000000000000 ) ) ;
#10329=CARTESIAN_POINT ( 'NONE',  ( 132.4999999999999432, -36.99999999999997868, -180.0000000000000000 ) ) ;
#10330=ORIENTED_EDGE ( 'NONE', *, *, #13299, .T. ) ;
#10333=LINE ( 'NONE', #13671, #4427 ) ;
#10336=AXIS2_PLACEMENT_3D ( 'NONE', #7825, #12120, #12260 ) ;
#10340=AXIS2_PLACEMENT_3D ( 'NONE', #9607, #14013, #5120 ) ;
#10349=ORIENTED_EDGE ( 'NONE', *, *, #8435, .F. ) ;
#10350=DIRECTION ( 'NONE',  ( 0.000000000000000000, 0.000000000000000000, -1.000000000000000000 ) ) ;
#10353=ORIENTED_EDGE ( 'NONE', *, *, #11185, .F. ) ;
#10356=VECTOR ( 'NONE', #9086, 1000.000000000000000 ) ;
#10357=FACE_OUTER_BOUND ( 'NONE', #14244, .T. ) ;
#10364=AXIS2_PLACEMENT_3D ( 'NONE', #3336, #3599, #11222 ) ;
#10366=VERTEX_POINT ( 'NONE', #12730 ) ;
#10367=ORIENTED_EDGE ( 'NONE', *, *, #1882, .T. ) ;
#10372=DIRECTION ( 'NONE',  ( 0.000000000000000000, 0.000000000000000000, 1.000000000000000000 ) ) ;
#10374=EDGE_LOOP ( 'NONE', ( #8477, #10441 ) ) ;
#10375=CARTESIAN_POINT ( 'NONE',  ( 119.9999999999999147, -225.0010000000000048, -169.9999999999999716 ) ) ;
#10378=CARTESIAN_POINT ( 'NONE',  ( 299.9999999999999432, -75.00000000000008527, 186.2999999999999829 ) ) ;
#10382=DIRECTION ( 'NONE',  ( -0.000000000000000000, -0.000000000000000000, -1.000000000000000000 ) ) ;
#10386=ORIENTED_EDGE ( 'NONE', *, *, #9968, .T. ) ;
#10387=ADVANCED_FACE ( 'NONE', ( #2206, #6633 ), #1025, .F. ) ;
#10391=DIRECTION ( 'NONE',  ( -0.000000000000000000, -0.000000000000000000, 1.000000000000000000 ) ) ;
#10393=VERTEX_POINT ( 'NONE', #5548 ) ;
#10397=FACE_OUTER_BOUND ( 'NONE', #14266, .T. ) ;
#10403=EDGE_CURVE ( 'NONE', #12400, #7986, #12082, .T. ) ;
#10404=DIRECTION ( 'NONE',  ( -1.000000000000000000, 0.000000000000000000, 0.000000000000000000 ) ) ;
#10405=CIRCLE ( 'NONE', #4393, 5.500000000000005329 ) ;
#10408=ORIENTED_EDGE ( 'NONE', *, *, #6997, .F. ) ;
#10411=CARTESIAN_POINT ( 'NONE',  ( 203.5000000000000000, -85.00000000000007105, 180.0000000000000000 ) ) ;
#10416=AXIS2_PLACEMENT_3D ( 'NONE', #1187, #3250, #1997 ) ;
#10418=DIRECTION ( 'NONE',  ( -0.000000000000000000, -0.000000000000000000, -1.000000000000000000 ) ) ;
#10425=CIRCLE ( 'NONE', #1138, 2.649999999999985700 ) ;
#10426=ORIENTED_EDGE ( 'NONE', *, *, #14207, .T. ) ;
#10437=CARTESIAN_POINT ( 'NONE',  ( 294.4999999999999432, -95.00000000000008527, -186.2999999999999829 ) ) ;
#10440=ORIENTED_EDGE ( 'NONE', *, *, #4414, .F. ) ;
#10441=ORIENTED_EDGE ( 'NONE', *, *, #3477, .F. ) ;
#10450=CIRCLE ( 'NONE', #2349, 2.649999999999985700 ) ;
#10453=VERTEX_POINT ( 'NONE', #3243 ) ;
#10457=LINE ( 'NONE', #7974, #2293 ) ;
#10458=AXIS2_PLACEMENT_3D ( 'NONE', #4108, #12019, #3173 ) ;
#10468=ORIENTED_EDGE ( 'NONE', *, *, #13753, .F. ) ;
#10471=CARTESIAN_POINT ( 'NONE',  ( 136.6666666666666288, -20.00000000000000000, -225.1500000000000625 ) ) ;
#10474=FACE_OUTER_BOUND ( 'NONE', #10806, .T. ) ;
#10497=DIRECTION ( 'NONE',  ( 0.000000000000000000, 0.000000000000000000, -1.000000000000000000 ) ) ;
#10499=DIRECTION ( 'NONE',  ( 0.000000000000000000, 1.000000000000000000, 0.000000000000000000 ) ) ;
#10507=DIRECTION ( 'NONE',  ( -0.8571673013836870192, 1.049727191973306873E-16, 0.5150380737757234151 ) ) ;
#10508=CARTESIAN_POINT ( 'NONE',  ( 0.000000000000000000, 0.000000000000000000, 0.000000000000000000 ) ) ;
#10511=LINE ( 'NONE', #1717, #8387 ) ;
#10516=ORIENTED_EDGE ( 'NONE', *, *, #871, .T. ) ;
#10518=ORIENTED_EDGE ( 'NONE', *, *, #3507, .F. ) ;
#10523=VERTEX_POINT ( 'NONE', #8520 ) ;
#10524=CARTESIAN_POINT ( 'NONE',  ( 142.6500000000000057, -95.00000000000008527, -190.0000000000000000 ) ) ;
#10530=EDGE_CURVE ( 'NONE', #10838, #11122, #8440, .T. ) ;
#10544=LINE ( 'NONE', #6260, #134 ) ;
#10545=CARTESIAN_POINT ( 'NONE',  ( 299.9999999999999432, -75.00000000000008527, 190.0000000000000000 ) ) ;
#10546=LINE ( 'NONE', #6050, #12201 ) ;
#10549=AXIS2_PLACEMENT_3D ( 'NONE', #7932, #7066, #2430 ) ;
#10550=FACE_OUTER_BOUND ( 'NONE', #5455, .T. ) ;
#10554=EDGE_CURVE ( 'NONE', #11518, #701, #5853, .T. ) ;
#10557=EDGE_CURVE ( 'NONE', #10366, #4959, #1696, .T. ) ;
#10558=VECTOR ( 'NONE', #4273, 1000.000000000000000 ) ;
#10563=VERTEX_POINT ( 'NONE', #7432 ) ;
#10589=AXIS2_PLACEMENT_3D ( 'NONE', #8305, #8224, #7149 ) ;
#10590=CIRCLE ( 'NONE', #9428, 2.649999999999985700 ) ;
#10591=ORIENTED_EDGE ( 'NONE', *, *, #716, .T. ) ;
#10598=DIRECTION ( 'NONE',  ( -0.000000000000000000, -0.000000000000000000, 1.000000000000000000 ) ) ;
#10608=VECTOR ( 'NONE', #11294, 1000.000000000000000 ) ;
#10613=DIRECTION ( 'NONE',  ( 1.000000000000000000, 0.000000000000000000, 0.000000000000000000 ) ) ;
#10614=AXIS2_PLACEMENT_3D ( 'NONE', #9304, #13717, #3790 ) ;
#10615=VERTEX_POINT ( 'NONE', #1920 ) ;
#10619=LINE ( 'NONE', #1678, #2139 ) ;
#10622=EDGE_LOOP ( 'NONE', ( #724, #3001, #10330, #12245 ) ) ;
#10624=ORIENTED_EDGE ( 'NONE', *, *, #3848, .F. ) ;
#10627=DIRECTION ( 'NONE',  ( 1.000000000000000000, 0.000000000000000000, 0.000000000000000000 ) ) ;
#10630=AXIS2_PLACEMENT_3D ( 'NONE', #10545, #5832, #577 ) ;
#10636=LINE ( 'NONE', #668, #8238 ) ;
#10639=CARTESIAN_POINT ( 'NONE',  ( 299.9999999999999432, -95.00000000000008527, -169.9999999999999716 ) ) ;
#10640=ORIENTED_EDGE ( 'NONE', *, *, #4457, .T. ) ;
#10648=EDGE_LOOP ( 'NONE', ( #5735, #8594 ) ) ;
#10649=CIRCLE ( 'NONE', #12959, 2.649999999999985700 ) ;
#10656=CARTESIAN_POINT ( 'NONE',  ( 203.5000000000000000, -85.00000000000007105, 180.0000000000000000 ) ) ;
#10657=CIRCLE ( 'NONE', #6252, 2.649999999999985700 ) ;
#10659=CARTESIAN_POINT ( 'NONE',  ( 305.4999999999999432, -75.00000000000008527, -186.2999999999999829 ) ) ;
#10663=CIRCLE ( 'NONE', #5856, 2.649999999999985700 ) ;
#10665=ORIENTED_EDGE ( 'NONE', *, *, #13504, .T. ) ;
#10668=DIRECTION ( 'NONE',  ( -1.000000000000000000, 0.000000000000000000, 0.000000000000000000 ) ) ;
#10681=CARTESIAN_POINT ( 'NONE',  ( 140.0000000000000000, -75.00000000000008527, -190.0000000000000000 ) ) ;
#10684=AXIS2_PLACEMENT_3D ( 'NONE', #10411, #2583, #13596 ) ;
#10689=VERTEX_POINT ( 'NONE', #7572 ) ;
#10695=EDGE_LOOP ( 'NONE', ( #8200, #845 ) ) ;
#10699=DIRECTION ( 'NONE',  ( 0.000000000000000000, 1.000000000000000000, 0.000000000000000000 ) ) ;
#10714=DIRECTION ( 'NONE',  ( -0.000000000000000000, 0.000000000000000000, 1.000000000000000000 ) ) ;
#10716=ORIENTED_EDGE ( 'NONE', *, *, #9788, .T. ) ;
#10718=DIRECTION ( 'NONE',  ( -0.000000000000000000, -0.000000000000000000, 1.000000000000000000 ) ) ;
#10722=LINE ( 'NONE', #9625, #7640 ) ;
#10737=CIRCLE ( 'NONE', #10030, 2.649999999999985700 ) ;
#10740=ORIENTED_EDGE ( 'NONE', *, *, #5173, .T. ) ;
#10762=CARTESIAN_POINT ( 'NONE',  ( 134.5000000000000000, -75.00000000000008527, -190.0000000000000000 ) ) ;
#10763=EDGE_CURVE ( 'NONE', #13552, #7639, #10737, .T. ) ;
#10767=EDGE_LOOP ( 'NONE', ( #12989, #5785, #9812 ) ) ;
#10769=CARTESIAN_POINT ( 'NONE',  ( 299.9999999999999432, -95.00000000000008527, -186.2999999999999829 ) ) ;
#10770=LINE ( 'NONE', #4384, #8745 ) ;
#10772=DIRECTION ( 'NONE',  ( -0.000000000000000000, -0.000000000000000000, 1.000000000000000000 ) ) ;
#10785=CARTESIAN_POINT ( 'NONE',  ( -30.00000000000002842, -225.0000000000000000, -169.9999999999999716 ) ) ;
#10787=EDGE_LOOP ( 'NONE', ( #10518, #5227, #3626, #10624 ) ) ;
#10788=DIRECTION ( 'NONE',  ( -0.000000000000000000, -0.000000000000000000, 1.000000000000000000 ) ) ;
#10792=EDGE_LOOP ( 'NONE', ( #12499, #4889 ) ) ;
#10795=CARTESIAN_POINT ( 'NONE',  ( 203.5000000000000000, -85.00000000000007105, 190.0000000000000000 ) ) ;
#10798=EDGE_CURVE ( 'NONE', #10296, #6403, #11188, .T. ) ;
#10802=CARTESIAN_POINT ( 'NONE',  ( -30.00000000000002842, -25.00000000000000000, 250.0000000000000000 ) ) ;
#10806=EDGE_LOOP ( 'NONE', ( #8699, #2201, #5355 ) ) ;
#10808=VECTOR ( 'NONE', #10507, 1000.000000000000000 ) ;
#10811=LINE ( 'NONE', #9648, #2792 ) ;
#10819=CIRCLE ( 'NONE', #12653, 2.649999999999985700 ) ;
#10833=DIRECTION ( 'NONE',  ( -1.000000000000000000, 0.000000000000000000, 0.000000000000000000 ) ) ;
#10837=DIRECTION ( 'NONE',  ( 1.000000000000000000, 0.000000000000000000, 0.000000000000000000 ) ) ;
#10838=VERTEX_POINT ( 'NONE', #2834 ) ;
#10841=AXIS2_PLACEMENT_3D ( 'NONE', #6619, #9008, #7840 ) ;
#10842=CARTESIAN_POINT ( 'NONE',  ( 299.9999999999999432, -75.00000000000008527, -190.0000000000000000 ) ) ;
#10845=CYLINDRICAL_SURFACE ( 'NONE', #228, 2.649999999999985700 ) ;
#10847=ADVANCED_FACE ( 'NONE', ( #630 ), #12688, .F. ) ;
#10849=CARTESIAN_POINT ( 'NONE',  ( 136.6666666666666288, -25.00000000000000000, -222.5000000000000853 ) ) ;
#10856=CARTESIAN_POINT ( 'NONE',  ( 140.0000000000000000, -75.00000000000008527, -169.9999999999999716 ) ) ;
#10860=ORIENTED_EDGE ( 'NONE', *, *, #5239, .T. ) ;
#10874=AXIS2_PLACEMENT_3D ( 'NONE', #12117, #1065, #8923 ) ;
#10881=DIRECTION ( 'NONE',  ( -0.000000000000000000, -0.000000000000000000, -1.000000000000000000 ) ) ;
#10884=DIRECTION ( 'NONE',  ( -0.000000000000000000, -0.000000000000000000, 1.000000000000000000 ) ) ;
#10886=ORIENTED_EDGE ( 'NONE', *, *, #2230, .F. ) ;
#10887=VECTOR ( 'NONE', #9839, 1000.000000000000000 ) ;
#10888=CARTESIAN_POINT ( 'NONE',  ( 307.5000000000000000, -36.99999999999997868, -169.9999999999999716 ) ) ;
#10891=EDGE_LOOP ( 'NONE', ( #11266, #6435, #5899, #4009 ) ) ;
#10895=CARTESIAN_POINT ( 'NONE',  ( -30.00000000000002842, -25.00000000000000000, 190.0000000000000000 ) ) ;
#10900=CARTESIAN_POINT ( 'NONE',  ( 134.9999999999999432, -56.99999999999997158, -180.0000000000000000 ) ) ;
#10903=DIRECTION ( 'NONE',  ( -1.000000000000000000, 0.000000000000000000, 0.000000000000000000 ) ) ;
#10905=ORIENTED_EDGE ( 'NONE', *, *, #11691, .T. ) ;
#10909=DIRECTION ( 'NONE',  ( -1.000000000000000000, 0.000000000000000000, 0.000000000000000000 ) ) ;
#10910=CARTESIAN_POINT ( 'NONE',  ( 302.5000000000000000, -56.99999999999997158, -169.9999999999999716 ) ) ;
#10911=DIRECTION ( 'NONE',  ( -0.000000000000000000, -0.000000000000000000, 1.000000000000000000 ) ) ;
#10916=ORIENTED_EDGE ( 'NONE', *, *, #10403, .F. ) ;
#10921=ORIENTED_EDGE ( 'NONE', *, *, #1602, .F. ) ;
#10922=DIRECTION ( 'NONE',  ( 1.000000000000000000, 0.000000000000000000, 0.000000000000000000 ) ) ;
#10926=DIRECTION ( 'NONE',  ( 1.000000000000000000, 0.000000000000000000, 0.000000000000000000 ) ) ;
#10929=CARTESIAN_POINT ( 'NONE',  ( 299.9999999999999432, -95.00000000000008527, 190.0000000000000000 ) ) ;
#10940=CARTESIAN_POINT ( 'NONE',  ( 294.4999999999999432, -75.00000000000008527, 190.0000000000000000 ) ) ;
#10944=ORIENTED_EDGE ( 'NONE', *, *, #10403, .T. ) ;
#10955=VECTOR ( 'NONE', #9168, 1000.000000000000000 ) ;
#10967=VERTEX_POINT ( 'NONE', #842 ) ;
#10968=DIRECTION ( 'NONE',  ( 1.000000000000000000, 0.000000000000000000, 0.000000000000000000 ) ) ;
#10970=CARTESIAN_POINT ( 'NONE',  ( 386.6666666666666288, -20.00000000000000000, 222.5000000000000853 ) ) ;
#10977=DIRECTION ( 'NONE',  ( 0.000000000000000000, 1.000000000000000000, 0.000000000000000000 ) ) ;
#10980=ORIENTED_EDGE ( 'NONE', *, *, #4544, .T. ) ;
#10985=CARTESIAN_POINT ( 'NONE',  ( 53.33333333333330017, -20.00000000000000000, -219.8500000000001080 ) ) ;
#10986=CARTESIAN_POINT ( 'NONE',  ( 236.4999999999999432, -85.00000000000007105, 180.0000000000000000 ) ) ;
#10995=CARTESIAN_POINT ( 'NONE',  ( 140.0000000000000000, -95.00000000000008527, -190.0000000000000000 ) ) ;
#11000=CARTESIAN_POINT ( 'NONE',  ( 305.0000000000000000, -56.99999999999997158, -181.5021515430661054 ) ) ;
#11001=CARTESIAN_POINT ( 'NONE',  ( 136.6666666666666288, -20.00000000000000000, 222.5000000000000853 ) ) ;
#11002=EDGE_CURVE ( 'NONE', #1558, #9645, #7934, .T. ) ;
#11004=ADVANCED_FACE ( 'NONE', ( #7466 ), #12907, .F. ) ;
#11011=EDGE_CURVE ( 'NONE', #1125, #10453, #6454, .T. ) ;
#11020=LINE ( 'NONE', #6451, #6847 ) ;
#11023=DIRECTION ( 'NONE',  ( -0.000000000000000000, -0.000000000000000000, -1.000000000000000000 ) ) ;
#11026=ORIENTED_EDGE ( 'NONE', *, *, #9596, .F. ) ;
#11029=EDGE_CURVE ( 'NONE', #5322, #3720, #7601, .T. ) ;
#11034=EDGE_CURVE ( 'NONE', #5038, #9120, #768, .T. ) ;
#11035=CARTESIAN_POINT ( 'NONE',  ( -30.00000000000002842, -225.0000000000000000, -169.9999999999999716 ) ) ;
#11040=DIRECTION ( 'NONE',  ( 0.000000000000000000, 1.000000000000000000, 0.000000000000000000 ) ) ;
#11044=CIRCLE ( 'NONE', #8518, 2.649999999999985700 ) ;
#11046=VERTEX_POINT ( 'NONE', #1876 ) ;
#11055=DIRECTION ( 'NONE',  ( -0.000000000000000000, 1.000000000000000000, -0.000000000000000000 ) ) ;
#11056=CIRCLE ( 'NONE', #8009, 5.500000000000005329 ) ;
#11058=SURFACE_SIDE_STYLE ('',( #7910 ) ) ;
#11061=VECTOR ( 'NONE', #11595, 1000.000000000000000 ) ;
#11071=DIRECTION ( 'NONE',  ( 0.000000000000000000, 0.000000000000000000, 1.000000000000000000 ) ) ;
#11075=AXIS2_PLACEMENT_3D ( 'NONE', #13200, #993, #14072 ) ;
#11076=CARTESIAN_POINT ( 'NONE',  ( 145.5000000000000284, -75.00000000000008527, 186.2999999999999829 ) ) ;
#11086=CARTESIAN_POINT ( 'NONE',  ( 136.6666666666666288, -20.00000000000000000, 219.8500000000001080 ) ) ;
#11090=EDGE_CURVE ( 'NONE', #634, #11403, #11899, .T. ) ;
#11094=CIRCLE ( 'NONE', #6689, 2.649999999999985700 ) ;
#11096=DIRECTION ( 'NONE',  ( -0.000000000000000000, -0.000000000000000000, 1.000000000000000000 ) ) ;
#11101=EDGE_LOOP ( 'NONE', ( #1605, #7051, #1048, #12387 ) ) ;
#11102=DIRECTION ( 'NONE',  ( -1.000000000000000000, 0.000000000000000000, 0.000000000000000000 ) ) ;
#11118=ORIENTED_EDGE ( 'NONE', *, *, #4827, .F. ) ;
#11120=LINE ( 'NONE', #14151, #7001 ) ;
#11122=VERTEX_POINT ( 'NONE', #8019 ) ;
#11124=ORIENTED_EDGE ( 'NONE', *, *, #9314, .F. ) ;
#11125=DIRECTION ( 'NONE',  ( 0.000000000000000000, 0.000000000000000000, -1.000000000000000000 ) ) ;
#11129=DIRECTION ( 'NONE',  ( -1.000000000000000000, 0.000000000000000000, 0.000000000000000000 ) ) ;
#11130=AXIS2_PLACEMENT_3D ( 'NONE', #1776, #816, #9702 ) ;
#11135=AXIS2_PLACEMENT_3D ( 'NONE', #2700, #7119, #13640 ) ;
#11140=AXIS2_PLACEMENT_3D ( 'NONE', #10795, #5145, #1933 ) ;
#11141=DIRECTION ( 'NONE',  ( -0.000000000000000000, -0.000000000000000000, -1.000000000000000000 ) ) ;
#11152=EDGE_LOOP ( 'NONE', ( #6092, #8937, #11950, #4394 ) ) ;
#11166=ORIENTED_EDGE ( 'NONE', *, *, #8678, .F. ) ;
#11167=EDGE_LOOP ( 'NONE', ( #6527, #7929, #9271, #9364 ) ) ;
#11171=FACE_BOUND ( 'NONE', #12008, .T. ) ;
#11176=DIRECTION ( 'NONE',  ( -1.000000000000000000, 0.000000000000000000, 0.000000000000000000 ) ) ;
#11185=EDGE_CURVE ( 'NONE', #3774, #3034, #14129, .T. ) ;
#11188=CIRCLE ( 'NONE', #13035, 2.649999999999985700 ) ;
#11193=AXIS2_PLACEMENT_3D ( 'NONE', #10769, #13872, #11998 ) ;
#11201=DIRECTION ( 'NONE',  ( 0.000000000000000000, 0.000000000000000000, -1.000000000000000000 ) ) ;
#11214=ADVANCED_FACE ( 'NONE', ( #7811 ), #4655, .F. ) ;
#11217=CARTESIAN_POINT ( 'NONE',  ( 140.0000000000000000, -75.00000000000008527, 190.0000000000000000 ) ) ;
#11220=DIRECTION ( 'NONE',  ( 0.8571673013836870192, 0.000000000000000000, 0.5150380737757234151 ) ) ;
#11221=DIRECTION ( 'NONE',  ( 0.000000000000000000, 0.000000000000000000, 1.000000000000000000 ) ) ;
#11222=DIRECTION ( 'NONE',  ( -1.000000000000000000, 0.000000000000000000, 0.000000000000000000 ) ) ;
#11223=VERTEX_POINT ( 'NONE', #4562 ) ;
#11225=CYLINDRICAL_SURFACE ( 'NONE', #13876, 5.500000000000005329 ) ;
#11231=EDGE_LOOP ( 'NONE', ( #8999, #7978 ) ) ;
#11235=EDGE_LOOP ( 'NONE', ( #4799, #2463, #10905 ) ) ;
#11236=DIRECTION ( 'NONE',  ( -0.000000000000000000, -0.000000000000000000, -1.000000000000000000 ) ) ;
#11245=ORIENTED_EDGE ( 'NONE', *, *, #12352, .T. ) ;
#11246=ORIENTED_EDGE ( 'NONE', *, *, #8161, .T. ) ;
#11255=CARTESIAN_POINT ( 'NONE',  ( 470.0000000000000000, -25.00000000000000000, -250.0000000000000000 ) ) ;
#11261=( NAMED_UNIT ( * ) PLANE_ANGLE_UNIT ( ) SI_UNIT ( $, .RADIAN. ) );
#11265=EDGE_LOOP ( 'NONE', ( #13303, #90, #2694, #9616 ) ) ;
#11266=ORIENTED_EDGE ( 'NONE', *, *, #13656, .F. ) ;
#11268=EDGE_LOOP ( 'NONE', ( #5057, #13780, #4991, #13413 ) ) ;
#11273=FACE_OUTER_BOUND ( 'NONE', #5821, .T. ) ;
#11275=EDGE_CURVE ( 'NONE', #10563, #8882, #12294, .T. ) ;
#11277=DIRECTION ( 'NONE',  ( 0.000000000000000000, 1.000000000000000000, 0.000000000000000000 ) ) ;
#11281=LINE ( 'NONE', #6921, #10955 ) ;
#11291=LINE ( 'NONE', #5561, #5360 ) ;
#11294=DIRECTION ( 'NONE',  ( -0.000000000000000000, -0.000000000000000000, -1.000000000000000000 ) ) ;
#11295=ORIENTED_EDGE ( 'NONE', *, *, #8718, .F. ) ;
#11296=CIRCLE ( 'NONE', #10364, 5.500000000000005329 ) ;
#11304=VERTEX_POINT ( 'NONE', #8097 ) ;
#11311=CARTESIAN_POINT ( 'NONE',  ( 299.9999999999999432, -75.00000000000008527, 186.2999999999999829 ) ) ;
#11313=DIRECTION ( 'NONE',  ( 1.000000000000000000, 0.000000000000000000, 0.000000000000000000 ) ) ;
#11325=VERTEX_POINT ( 'NONE', #9411 ) ;
#11327=ORIENTED_EDGE ( 'NONE', *, *, #7456, .F. ) ;
#11328=AXIS2_PLACEMENT_3D ( 'NONE', #11597, #5084, #691 ) ;
#11338=DIRECTION ( 'NONE',  ( -0.000000000000000000, -0.000000000000000000, 1.000000000000000000 ) ) ;
#11339=VERTEX_POINT ( 'NONE', #9485 ) ;
#11349=VECTOR ( 'NONE', #1186, 1000.000000000000000 ) ;
#11351=AXIS2_PLACEMENT_3D ( 'NONE', #11001, #4407, #5481 ) ;
#11352=DIRECTION ( 'NONE',  ( -0.000000000000000000, -0.000000000000000000, -1.000000000000000000 ) ) ;
#11354=AXIS2_PLACEMENT_3D ( 'NONE', #5613, #2130, #6559 ) ;
#11360=DIRECTION ( 'NONE',  ( 1.000000000000000000, 0.000000000000000000, 0.000000000000000000 ) ) ;
#11363=CIRCLE ( 'NONE', #2339, 5.500000000000005329 ) ;
#11370=AXIS2_PLACEMENT_3D ( 'NONE', #2576, #9464, #6993 ) ;
#11373=VERTEX_POINT ( 'NONE', #2890 ) ;
#11378=CYLINDRICAL_SURFACE ( 'NONE', #828, 5.500000000000005329 ) ;
#11388=CARTESIAN_POINT ( 'NONE',  ( 386.6666666666666288, -20.00000000000000000, 222.5000000000000853 ) ) ;
#11390=CIRCLE ( 'NONE', #1874, 2.500000000000002220 ) ;
#11398=FACE_OUTER_BOUND ( 'NONE', #7363, .T. ) ;
#11400=CYLINDRICAL_SURFACE ( 'NONE', #1286, 10.00000000000000888 ) ;
#11403=VERTEX_POINT ( 'NONE', #5146 ) ;
#11405=DIRECTION ( 'NONE',  ( 0.000000000000000000, 0.000000000000000000, 1.000000000000000000 ) ) ;
#11411=ORIENTED_EDGE ( 'NONE', *, *, #13899, .F. ) ;
#11423=CARTESIAN_POINT ( 'NONE',  ( 299.9999999999999432, -95.00000000000008527, 169.9999999999999716 ) ) ;
#11431=DIRECTION ( 'NONE',  ( -0.000000000000000000, -0.000000000000000000, 1.000000000000000000 ) ) ;
#11434=DIRECTION ( 'NONE',  ( -0.000000000000000000, 1.000000000000000000, -0.000000000000000000 ) ) ;
#11436=DIRECTION ( 'NONE',  ( 0.000000000000000000, 0.000000000000000000, -1.000000000000000000 ) ) ;
#11443=EDGE_CURVE ( 'NONE', #7589, #4114, #5424, .T. ) ;
#11444=ORIENTED_EDGE ( 'NONE', *, *, #6248, .T. ) ;
#11445=DIRECTION ( 'NONE',  ( -0.000000000000000000, -0.000000000000000000, -1.000000000000000000 ) ) ;
#11448=EDGE_CURVE ( 'NONE', #11751, #5872, #9563, .T. ) ;
#11450=ADVANCED_FACE ( 'NONE', ( #1862, #11735 ), #6285, .F. ) ;
#11451=CARTESIAN_POINT ( 'NONE',  ( 134.9999999999999432, -36.99999999999997868, -181.5021515430661054 ) ) ;
#11458=DIRECTION ( 'NONE',  ( 1.000000000000000000, 0.000000000000000000, 0.000000000000000000 ) ) ;
#11463=CIRCLE ( 'NONE', #7061, 2.500000000000002220 ) ;
#11466=EDGE_CURVE ( 'NONE', #5335, #11791, #10212, .T. ) ;
#11467=FACE_OUTER_BOUND ( 'NONE', #10044, .T. ) ;
#11476=FACE_BOUND ( 'NONE', #8638, .T. ) ;
#11485=LINE ( 'NONE', #5977, #6865 ) ;
#11486=AXIS2_PLACEMENT_3D ( 'NONE', #13922, #5016, #6024 ) ;
#11487=LINE ( 'NONE', #6120, #3224 ) ;
#11491=CARTESIAN_POINT ( 'NONE',  ( 134.9999999999999432, -56.99999999999997158, -180.0000000000000000 ) ) ;
#11492=DIRECTION ( 'NONE',  ( -0.000000000000000000, -0.000000000000000000, 1.000000000000000000 ) ) ;
#11506=DIRECTION ( 'NONE',  ( -0.000000000000000000, -0.000000000000000000, -1.000000000000000000 ) ) ;
#11507=CIRCLE ( 'NONE', #10109, 2.649999999999985700 ) ;
#11510=FACE_OUTER_BOUND ( 'NONE', #196, .T. ) ;
#11515=EDGE_CURVE ( 'NONE', #6665, #5470, #2002, .T. ) ;
#11516=AXIS2_PLACEMENT_3D ( 'NONE', #10375, #2472, #6897 ) ;
#11518=VERTEX_POINT ( 'NONE', #10196 ) ;
#11522=CARTESIAN_POINT ( 'NONE',  ( 386.6666666666666288, -20.00000000000000000, -222.5000000000000853 ) ) ;
#11526=FACE_OUTER_BOUND ( 'NONE', #4741, .T. ) ;
#11529=ORIENTED_EDGE ( 'NONE', *, *, #8902, .F. ) ;
#11530=ORIENTED_EDGE ( 'NONE', *, *, #6117, .F. ) ;
#11532=ORIENTED_EDGE ( 'NONE', *, *, #5065, .F. ) ;
#11534=DIRECTION ( 'NONE',  ( -0.000000000000000000, 0.000000000000000000, 1.000000000000000000 ) ) ;
#11536=AXIS2_PLACEMENT_3D ( 'NONE', #11958, #12895, #2972 ) ;
#11538=DIRECTION ( 'NONE',  ( 0.8571673013836870192, 0.000000000000000000, 0.5150380737757234151 ) ) ;
#11539=EDGE_LOOP ( 'NONE', ( #1724, #13811 ) ) ;
#11543=ORIENTED_EDGE ( 'NONE', *, *, #10763, .F. ) ;
#11549=VERTEX_POINT ( 'NONE', #11086 ) ;
#11552=VERTEX_POINT ( 'NONE', #4485 ) ;
#11554=VECTOR ( 'NONE', #8546, 1000.000000000000000 ) ;
#11560=CARTESIAN_POINT ( 'NONE',  ( 236.4999999999999432, -85.00000000000007105, 180.0000000000000000 ) ) ;
#11563=FACE_OUTER_BOUND ( 'NONE', #8795, .T. ) ;
#11567=EDGE_CURVE ( 'NONE', #11339, #14007, #6961, .T. ) ;
#11569=VERTEX_POINT ( 'NONE', #8963 ) ;
#11570=ORIENTED_EDGE ( 'NONE', *, *, #7868, .F. ) ;
#11571=CARTESIAN_POINT ( 'NONE',  ( -30.00000000000002842, -25.00000000000000000, 250.0000000000000000 ) ) ;
#11575=EDGE_CURVE ( 'NONE', #12771, #3344, #11291, .T. ) ;
#11578=CARTESIAN_POINT ( 'NONE',  ( 142.6500000000000057, -95.00000000000008527, -186.2999999999999829 ) ) ;
#11582=AXIS2_PLACEMENT_3D ( 'NONE', #7230, #2888, #11662 ) ;
#11595=DIRECTION ( 'NONE',  ( -0.000000000000000000, -0.000000000000000000, 1.000000000000000000 ) ) ;
#11597=CARTESIAN_POINT ( 'NONE',  ( 305.0000000000000000, -36.99999999999997868, -180.0000000000000000 ) ) ;
#11606=ORIENTED_EDGE ( 'NONE', *, *, #3817, .F. ) ;
#11607=CARTESIAN_POINT ( 'NONE',  ( 319.9999999999999432, -24.99999999999999289, -19.99999999999998934 ) ) ;
#11609=AXIS2_PLACEMENT_3D ( 'NONE', #7064, #8214, #511 ) ;
#11610=CYLINDRICAL_SURFACE ( 'NONE', #6150, 2.649999999999985700 ) ;
#11620=CYLINDRICAL_SURFACE ( 'NONE', #4115, 2.500000000000002220 ) ;
#11621=EDGE_CURVE ( 'NONE', #1677, #14253, #1189, .T. ) ;
#11626=LINE ( 'NONE', #10762, #7427 ) ;
#11627=VECTOR ( 'NONE', #8031, 1000.000000000000000 ) ;
#11628=VECTOR ( 'NONE', #4275, 1000.000000000000000 ) ;
#11632=FACE_OUTER_BOUND ( 'NONE', #1573, .T. ) ;
#11638=DIRECTION ( 'NONE',  ( 1.000000000000000000, 0.000000000000000000, 0.000000000000000000 ) ) ;
#11639=CARTESIAN_POINT ( 'NONE',  ( 305.4999999999999432, -95.00000000000008527, -190.0000000000000000 ) ) ;
#11640=EDGE_CURVE ( 'NONE', #5038, #3114, #13250, .T. ) ;
#11641=CARTESIAN_POINT ( 'NONE',  ( 299.9999999999999432, -75.00000000000008527, 190.0000000000000000 ) ) ;
#11648=FACE_OUTER_BOUND ( 'NONE', #7141, .T. ) ;
#11650=EDGE_CURVE ( 'NONE', #13280, #2338, #8827, .T. ) ;
#11655=CARTESIAN_POINT ( 'NONE',  ( 140.0000000000000000, -75.00000000000008527, -186.2999999999999829 ) ) ;
#11657=FACE_OUTER_BOUND ( 'NONE', #4370, .T. ) ;
#11660=DIRECTION ( 'NONE',  ( 0.000000000000000000, 1.000000000000000000, 0.000000000000000000 ) ) ;
#11662=DIRECTION ( 'NONE',  ( 1.000000000000000000, 0.000000000000000000, 0.000000000000000000 ) ) ;
#11665=LINE ( 'NONE', #3690, #7096 ) ;
#11680=DIRECTION ( 'NONE',  ( 0.000000000000000000, 0.000000000000000000, 1.000000000000000000 ) ) ;
#11682=DIRECTION ( 'NONE',  ( 0.000000000000000000, 1.000000000000000000, 0.000000000000000000 ) ) ;
#11686=FACE_BOUND ( 'NONE', #3637, .T. ) ;
#11688=FACE_OUTER_BOUND ( 'NONE', #12930, .T. ) ;
#11691=EDGE_CURVE ( 'NONE', #5470, #8094, #2572, .T. ) ;
#11697=ORIENTED_EDGE ( 'NONE', *, *, #3049, .T. ) ;
#11699=ORIENTED_EDGE ( 'NONE', *, *, #9972, .T. ) ;
#11708=CARTESIAN_POINT ( 'NONE',  ( 203.5000000000000000, -85.00000000000007105, 180.0000000000000000 ) ) ;
#11712=ORIENTED_EDGE ( 'NONE', *, *, #2055, .F. ) ;
#11715=AXIS2_PLACEMENT_3D ( 'NONE', #12981, #7392, #8551 ) ;
#11717=DIRECTION ( 'NONE',  ( 0.000000000000000000, 1.000000000000000000, 0.000000000000000000 ) ) ;
#11718=EDGE_CURVE ( 'NONE', #9107, #9676, #10333, .T. ) ;
#11719=DIRECTION ( 'NONE',  ( 1.000000000000000000, 0.000000000000000000, 0.000000000000000000 ) ) ;
#11721=DIRECTION ( 'NONE',  ( -0.000000000000000000, 0.000000000000000000, 1.000000000000000000 ) ) ;
#11725=FACE_OUTER_BOUND ( 'NONE', #6612, .T. ) ;
#11729=ADVANCED_FACE ( 'NONE', ( #11648 ), #8002, .F. ) ;
#11731=EDGE_CURVE ( 'NONE', #6238, #4007, #5842, .T. ) ;
#11732=EDGE_LOOP ( 'NONE', ( #2901, #8409 ) ) ;
#11735=FACE_OUTER_BOUND ( 'NONE', #12424, .T. ) ;
#11736=AXIS2_PLACEMENT_3D ( 'NONE', #3338, #7735, #9243 ) ;
#11737=ORIENTED_EDGE ( 'NONE', *, *, #9735, .F. ) ;
#11751=VERTEX_POINT ( 'NONE', #2729 ) ;
#11762=ORIENTED_EDGE ( 'NONE', *, *, #4954, .F. ) ;
#11770=ORIENTED_EDGE ( 'NONE', *, *, #6144, .F. ) ;
#11778=ORIENTED_EDGE ( 'NONE', *, *, #11275, .F. ) ;
#11791=VERTEX_POINT ( 'NONE', #1473 ) ;
#11792=DIRECTION ( 'NONE',  ( 1.000000000000000000, 0.000000000000000000, 0.000000000000000000 ) ) ;
#11801=ADVANCED_FACE ( 'NONE', ( #2802 ), #6737, .F. ) ;
#11802=VERTEX_POINT ( 'NONE', #295 ) ;
#11811=EDGE_CURVE ( 'NONE', #3034, #3774, #5817, .T. ) ;
#11816=VECTOR ( 'NONE', #5069, 1000.000000000000000 ) ;
#11817=ADVANCED_FACE ( 'NONE', ( #13743 ), #9109, .F. ) ;
#11822=EDGE_LOOP ( 'NONE', ( #2039, #1028 ) ) ;
#11832=EDGE_LOOP ( 'NONE', ( #805, #4465, #10426 ) ) ;
#11833=CARTESIAN_POINT ( 'NONE',  ( 299.9999999999999432, -95.00000000000008527, -186.2999999999999829 ) ) ;
#11836=CARTESIAN_POINT ( 'NONE',  ( 53.33333333333330017, -25.00000000000000000, -222.5000000000000853 ) ) ;
#11852=DIRECTION ( 'NONE',  ( 0.000000000000000000, 1.000000000000000000, 0.000000000000000000 ) ) ;
#11854=DIRECTION ( 'NONE',  ( 1.000000000000000000, 0.000000000000000000, 0.000000000000000000 ) ) ;
#11860=DIRECTION ( 'NONE',  ( -1.000000000000000000, 0.000000000000000000, 0.000000000000000000 ) ) ;
#11869=FACE_BOUND ( 'NONE', #5185, .T. ) ;
#11870=ORIENTED_EDGE ( 'NONE', *, *, #1056, .T. ) ;
#11872=FACE_OUTER_BOUND ( 'NONE', #8166, .T. ) ;
#11878=EDGE_LOOP ( 'NONE', ( #1658, #11570, #6957, #9532 ) ) ;
#11882=CIRCLE ( 'NONE', #1202, 2.649999999999985700 ) ;
#11888=CARTESIAN_POINT ( 'NONE',  ( 53.33333333333330017, -25.00000000000000000, 219.8500000000001080 ) ) ;
#11891=LINE ( 'NONE', #10802, #8524 ) ;
#11892=DIRECTION ( 'NONE',  ( 0.000000000000000000, 0.000000000000000000, 1.000000000000000000 ) ) ;
#11899=LINE ( 'NONE', #1945, #9521 ) ;
#11910=CARTESIAN_POINT ( 'NONE',  ( 386.6666666666666288, -25.00000000000000000, -222.5000000000000853 ) ) ;
#11916=VERTEX_POINT ( 'NONE', #6423 ) ;
#11917=EDGE_CURVE ( 'NONE', #3111, #1839, #11507, .T. ) ;
#11918=ADVANCED_FACE ( 'NONE', ( #4175 ), #881, .F. ) ;
#11925=ORIENTED_EDGE ( 'NONE', *, *, #4301, .F. ) ;
#11929=PLANE ( 'NONE',  #7543 ) ;
#11942=FACE_BOUND ( 'NONE', #2057, .T. ) ;
#11943=CIRCLE ( 'NONE', #10549, 5.500000000000005329 ) ;
#11945=DIRECTION ( 'NONE',  ( -1.000000000000000000, 0.000000000000000000, 0.000000000000000000 ) ) ;
#11946=EDGE_CURVE ( 'NONE', #1416, #9015, #10636, .T. ) ;
#11949=DIRECTION ( 'NONE',  ( 0.000000000000000000, 0.000000000000000000, -1.000000000000000000 ) ) ;
#11950=ORIENTED_EDGE ( 'NONE', *, *, #12706, .F. ) ;
#11952=VERTEX_POINT ( 'NONE', #5132 ) ;
#11956=CYLINDRICAL_SURFACE ( 'NONE', #6642, 2.649999999999985700 ) ;
#11958=CARTESIAN_POINT ( 'NONE',  ( 134.9999999999999432, -56.99999999999997158, -169.9999999999999716 ) ) ;
#11963=CARTESIAN_POINT ( 'NONE',  ( -30.00000000000002842, -225.0000000000000000, -190.0000000000000000 ) ) ;
#11972=DIRECTION ( 'NONE',  ( -0.000000000000000000, 1.000000000000000000, -0.000000000000000000 ) ) ;
#11977=FACE_OUTER_BOUND ( 'NONE', #5192, .T. ) ;
#11978=VECTOR ( 'NONE', #12579, 1000.000000000000000 ) ;
#11984=ORIENTED_EDGE ( 'NONE', *, *, #5091, .F. ) ;
#11985=ORIENTED_EDGE ( 'NONE', *, *, #5065, .T. ) ;
#11992=ORIENTED_EDGE ( 'NONE', *, *, #3564, .F. ) ;
#11994=ORIENTED_EDGE ( 'NONE', *, *, #434, .F. ) ;
#11996=AXIS2_PLACEMENT_3D ( 'NONE', #267, #1447, #9217 ) ;
#11997=AXIS2_PLACEMENT_3D ( 'NONE', #10378, #6025, #9145 ) ;
#11998=DIRECTION ( 'NONE',  ( -1.000000000000000000, 0.000000000000000000, 0.000000000000000000 ) ) ;
#11999=LINE ( 'NONE', #5257, #4801 ) ;
#12001=ADVANCED_FACE ( 'NONE', ( #8740 ), #1101, .F. ) ;
#12006=CONICAL_SURFACE ( 'NONE', #14069, 2.500000000000002220, 1.029744260000002631 ) ;
#12008=EDGE_LOOP ( 'NONE', ( #8281, #7236 ) ) ;
#12009=CIRCLE ( 'NONE', #13264, 2.649999999999985700 ) ;
#12017=VECTOR ( 'NONE', #6261, 1000.000000000000000 ) ;
#12019=DIRECTION ( 'NONE',  ( -0.000000000000000000, -0.000000000000000000, 1.000000000000000000 ) ) ;
#12022=DIRECTION ( 'NONE',  ( -0.000000000000000000, -1.000000000000000000, -0.000000000000000000 ) ) ;
#12023=EDGE_LOOP ( 'NONE', ( #8437, #1828 ) ) ;
#12030=CARTESIAN_POINT ( 'NONE',  ( 299.9999999999999432, -75.00000000000008527, -190.0000000000000000 ) ) ;
#12035=ORIENTED_EDGE ( 'NONE', *, *, #8445, .T. ) ;
#12036=FACE_OUTER_BOUND ( 'NONE', #647, .T. ) ;
#12041=VERTEX_POINT ( 'NONE', #8950 ) ;
#12042=VERTEX_POINT ( 'NONE', #2205 ) ;
#12044=DIRECTION ( 'NONE',  ( 1.000000000000000000, 0.000000000000000000, 0.000000000000000000 ) ) ;
#12060=LINE ( 'NONE', #4443, #9378 ) ;
#12061=VERTEX_POINT ( 'NONE', #13367 ) ;
#12062=CARTESIAN_POINT ( 'NONE',  ( 386.6666666666666288, -25.00000000000000000, -219.8500000000001080 ) ) ;
#12070=DIRECTION ( 'NONE',  ( -0.000000000000000000, -0.000000000000000000, 1.000000000000000000 ) ) ;
#12071=EDGE_CURVE ( 'NONE', #7265, #8495, #8952, .T. ) ;
#12082=LINE ( 'NONE', #5, #10259 ) ;
#12085=EDGE_CURVE ( 'NONE', #4114, #3377, #4532, .T. ) ;
#12087=LINE ( 'NONE', #4324, #3674 ) ;
#12094=EDGE_CURVE ( 'NONE', #2563, #11122, #832, .T. ) ;
#12097=DIRECTION ( 'NONE',  ( 1.000000000000000000, 0.000000000000000000, 0.000000000000000000 ) ) ;
#12098=EDGE_CURVE ( 'NONE', #12042, #6338, #11056, .T. ) ;
#12100=CIRCLE ( 'NONE', #2376, 5.500000000000005329 ) ;
#12101=CARTESIAN_POINT ( 'NONE',  ( 119.9999999999999147, -24.99999999999999289, 19.99999999999998934 ) ) ;
#12105=CARTESIAN_POINT ( 'NONE',  ( 469.9999999999998863, -225.0000000000000000, 190.0000000000000000 ) ) ;
#12110=CARTESIAN_POINT ( 'NONE',  ( 140.0000000000000000, -95.00000000000008527, 190.0000000000000000 ) ) ;
#12114=CARTESIAN_POINT ( 'NONE',  ( 140.0000000000000000, -95.00000000000008527, 186.2999999999999829 ) ) ;
#12115=CARTESIAN_POINT ( 'NONE',  ( -30.00000000000002842, -20.00000000000000000, -250.0000000000000000 ) ) ;
#12117=CARTESIAN_POINT ( 'NONE',  ( 136.6666666666666288, -20.00000000000000000, -222.5000000000000853 ) ) ;
#12120=DIRECTION ( 'NONE',  ( -0.000000000000000000, -0.000000000000000000, 1.000000000000000000 ) ) ;
#12126=DIRECTION ( 'NONE',  ( -0.000000000000000000, 1.000000000000000000, -0.000000000000000000 ) ) ;
#12127=ORIENTED_EDGE ( 'NONE', *, *, #2035, .T. ) ;
#12133=DIRECTION ( 'NONE',  ( -1.000000000000000000, 0.000000000000000000, -0.000000000000000000 ) ) ;
#12136=CARTESIAN_POINT ( 'NONE',  ( 219.9999999999999716, -85.00000000000007105, -250.0009999999999764 ) ) ;
#12143=VERTEX_POINT ( 'NONE', #4 ) ;
#12155=DIRECTION ( 'NONE',  ( -0.000000000000000000, -0.000000000000000000, 1.000000000000000000 ) ) ;
#12170=EDGE_LOOP ( 'NONE', ( #1680, #2306, #279 ) ) ;
#12175=VECTOR ( 'NONE', #9046, 1000.000000000000000 ) ;
#12178=CARTESIAN_POINT ( 'NONE',  ( 297.3499999999999659, -75.00000000000008527, -190.0000000000000000 ) ) ;
#12182=CARTESIAN_POINT ( 'NONE',  ( 119.9999999999999147, -225.0010000000000048, 169.9999999999999716 ) ) ;
#12196=EDGE_LOOP ( 'NONE', ( #5634, #13865, #10860, #1742 ) ) ;
#12201=VECTOR ( 'NONE', #13873, 1000.000000000000000 ) ;
#12203=CARTESIAN_POINT ( 'NONE',  ( 219.9999999999999716, -20.00000000000000000, -222.5000000000000853 ) ) ;
#12206=DIRECTION ( 'NONE',  ( 0.000000000000000000, 0.000000000000000000, -1.000000000000000000 ) ) ;
#12208=VERTEX_POINT ( 'NONE', #4892 ) ;
#12211=VECTOR ( 'NONE', #1009, 1000.000000000000000 ) ;
#12215=EDGE_LOOP ( 'NONE', ( #13674, #11166 ) ) ;
#12219=AXIS2_PLACEMENT_3D ( 'NONE', #10849, #7637, #1095 ) ;
#12223=CARTESIAN_POINT ( 'NONE',  ( -30.00000000000002842, -25.00000000000000000, 250.0000000000000000 ) ) ;
#12225=AXIS2_PLACEMENT_3D ( 'NONE', #7176, #14066, #7472 ) ;
#12239=CARTESIAN_POINT ( 'NONE',  ( 140.0000000000000000, -75.00000000000008527, 190.0000000000000000 ) ) ;
#12241=EDGE_CURVE ( 'NONE', #6402, #9645, #2568, .T. ) ;
#12245=ORIENTED_EDGE ( 'NONE', *, *, #13580, .T. ) ;
#12253=CARTESIAN_POINT ( 'NONE',  ( 302.5000000000000000, -36.99999999999997868, -180.0000000000000000 ) ) ;
#12256=AXIS2_PLACEMENT_3D ( 'NONE', #11388, #9205, #2611 ) ;
#12258=DIRECTION ( 'NONE',  ( -0.000000000000000000, 1.000000000000000000, -0.000000000000000000 ) ) ;
#12260=DIRECTION ( 'NONE',  ( 1.000000000000000000, 0.000000000000000000, 0.000000000000000000 ) ) ;
#12281=SHAPE_REPRESENTATION_RELATIONSHIP ( 'NONE' , 'NONE' ,  #2740, #12845 ) ;
#12284=DIRECTION ( 'NONE',  ( -0.8571673013836870192, 1.049727191973306873E-16, 0.5150380737757234151 ) ) ;
#12285=ORIENTED_EDGE ( 'NONE', *, *, #8416, .T. ) ;
#12288=AXIS2_PLACEMENT_3D ( 'NONE', #14142, #9518, #8644 ) ;
#12291=CARTESIAN_POINT ( 'NONE',  ( 386.6666666666666288, -20.00000000000000000, 222.5000000000000853 ) ) ;
#12294=CIRCLE ( 'NONE', #12748, 5.500000000000005329 ) ;
#12299=DIRECTION ( 'NONE',  ( -0.000000000000000000, -0.000000000000000000, 1.000000000000000000 ) ) ;
#12307=CARTESIAN_POINT ( 'NONE',  ( 294.4999999999999432, -75.00000000000008527, 190.0000000000000000 ) ) ;
#12317=ORIENTED_EDGE ( 'NONE', *, *, #11275, .T. ) ;
#12327=FACE_OUTER_BOUND ( 'NONE', #9759, .T. ) ;
#12336=EDGE_LOOP ( 'NONE', ( #12761, #7765 ) ) ;
#12338=EDGE_CURVE ( 'NONE', #2338, #13280, #3189, .T. ) ;
#12341=ORIENTED_EDGE ( 'NONE', *, *, #2918, .T. ) ;
#12345=VERTEX_POINT ( 'NONE', #6005 ) ;
#12349=PLANE ( 'NONE',  #4404 ) ;
#12352=EDGE_CURVE ( 'NONE', #8359, #14256, #14058, .T. ) ;
#12353=EDGE_CURVE ( 'NONE', #6756, #8236, #8020, .T. ) ;
#12354=FACE_BOUND ( 'NONE', #6631, .T. ) ;
#12358=EDGE_CURVE ( 'NONE', #11122, #2563, #363, .T. ) ;
#12387=ORIENTED_EDGE ( 'NONE', *, *, #2224, .F. ) ;
#12394=DIRECTION ( 'NONE',  ( 1.000000000000000000, 0.000000000000000000, 0.000000000000000000 ) ) ;
#12400=VERTEX_POINT ( 'NONE', #5324 ) ;
#12407=DIRECTION ( 'NONE',  ( -0.000000000000000000, -1.000000000000000000, -0.000000000000000000 ) ) ;
#12410=CARTESIAN_POINT ( 'NONE',  ( 140.0000000000000000, -75.00000000000008527, -190.0000000000000000 ) ) ;
#12417=FACE_BOUND ( 'NONE', #9880, .T. ) ;
#12420=AXIS2_PLACEMENT_3D ( 'NONE', #2109, #4224, #14077 ) ;
#12421=ORIENTED_EDGE ( 'NONE', *, *, #10092, .T. ) ;
#12424=EDGE_LOOP ( 'NONE', ( #2725, #8312 ) ) ;
#12435=DIRECTION ( 'NONE',  ( -1.000000000000000000, 0.000000000000000000, 0.000000000000000000 ) ) ;
#12436=AXIS2_PLACEMENT_3D ( 'NONE', #9337, #11434, #5847 ) ;
#12437=DIRECTION ( 'NONE',  ( 0.000000000000000000, 0.000000000000000000, -1.000000000000000000 ) ) ;
#12440=ORIENTED_EDGE ( 'NONE', *, *, #9608, .F. ) ;
#12443=AXIS2_PLACEMENT_3D ( 'NONE', #942, #5404, #12206 ) ;
#12450=AXIS2_PLACEMENT_3D ( 'NONE', #8188, #12407, #1297 ) ;
#12451=AXIS2_PLACEMENT_3D ( 'NONE', #991, #5651, #5582 ) ;
#12452=DIRECTION ( 'NONE',  ( -1.000000000000000000, 0.000000000000000000, 0.000000000000000000 ) ) ;
#12454=CARTESIAN_POINT ( 'NONE',  ( 303.3333333333333144, -20.00000000000000000, -222.5000000000000853 ) ) ;
#12459=AXIS2_PLACEMENT_3D ( 'NONE', #10785, #10714, #13965 ) ;
#12461=EDGE_LOOP ( 'NONE', ( #5071, #5425, #7605, #751 ) ) ;
#12469=CARTESIAN_POINT ( 'NONE',  ( 302.6499999999999204, -95.00000000000008527, 190.0000000000000000 ) ) ;
#12474=EDGE_CURVE ( 'NONE', #5437, #9413, #8253, .T. ) ;
#12478=CARTESIAN_POINT ( 'NONE',  ( 134.5000000000000000, -95.00000000000008527, -190.0000000000000000 ) ) ;
#12480=PLANE ( 'NONE',  #11516 ) ;
#12485=DIRECTION ( 'NONE',  ( 0.000000000000000000, 0.000000000000000000, 1.000000000000000000 ) ) ;
#12489=LINE ( 'NONE', #8057, #10356 ) ;
#12494=ORIENTED_EDGE ( 'NONE', *, *, #614, .T. ) ;
#12495=DIRECTION ( 'NONE',  ( -0.000000000000000000, -1.000000000000000000, -0.000000000000000000 ) ) ;
#12497=ORIENTED_EDGE ( 'NONE', *, *, #11029, .F. ) ;
#12499=ORIENTED_EDGE ( 'NONE', *, *, #9393, .F. ) ;
#12507=CIRCLE ( 'NONE', #2316, 5.500000000000005329 ) ;
#12509=CARTESIAN_POINT ( 'NONE',  ( 119.9999999999999147, -24.99999999999999289, -169.9999999999999716 ) ) ;
#12517=EDGE_CURVE ( 'NONE', #8094, #8759, #2120, .T. ) ;
#12521=EDGE_CURVE ( 'NONE', #11569, #8359, #122, .T. ) ;
#12522=CARTESIAN_POINT ( 'NONE',  ( 297.3499999999999659, -75.00000000000008527, 186.2999999999999829 ) ) ;
#12523=CYLINDRICAL_SURFACE ( 'NONE', #9482, 2.649999999999985700 ) ;
#12525=AXIS2_PLACEMENT_3D ( 'NONE', #7003, #11431, #1404 ) ;
#12530=STYLED_ITEM('',(#14389),#3574);
#12535=VECTOR ( 'NONE', #11277, 1000.000000000000000 ) ;
#12536=ORIENTED_EDGE ( 'NONE', *, *, #13435, .T. ) ;
#12542=CARTESIAN_POINT ( 'NONE',  ( 142.6500000000000057, -75.00000000000008527, -169.9999999999999716 ) ) ;
#12551=ORIENTED_EDGE ( 'NONE', *, *, #11090, .T. ) ;
#12554=CARTESIAN_POINT ( 'NONE',  ( 307.5000000000000000, -36.99999999999997868, -180.0000000000000000 ) ) ;
#12555=ORIENTED_EDGE ( 'NONE', *, *, #4954, .T. ) ;
#12557=DIRECTION ( 'NONE',  ( -1.000000000000000000, 0.000000000000000000, 0.000000000000000000 ) ) ;
#12559=ORIENTED_EDGE ( 'NONE', *, *, #530, .T. ) ;
#12565=FACE_BOUND ( 'NONE', #10792, .T. ) ;
#12567=ORIENTED_EDGE ( 'NONE', *, *, #3564, .T. ) ;
#12579=DIRECTION ( 'NONE',  ( 0.000000000000000000, 1.000000000000000000, 0.000000000000000000 ) ) ;
#12586=EDGE_LOOP ( 'NONE', ( #3259, #3558, #5857, #3559 ) ) ;
#12590=VERTEX_POINT ( 'NONE', #6550 ) ;
#12591=FACE_OUTER_BOUND ( 'NONE', #4958, .T. ) ;
#12599=CARTESIAN_POINT ( 'NONE',  ( -30.00000000000002842, -25.00000000000000000, -169.9999999999999716 ) ) ;
#12614=ORIENTED_EDGE ( 'NONE', *, *, #4592, .F. ) ;
#12616=CARTESIAN_POINT ( 'NONE',  ( 229.9999999999999716, -85.00000000000007105, -250.0009999999999764 ) ) ;
#12624=ORIENTED_EDGE ( 'NONE', *, *, #13192, .T. ) ;
#12628=CARTESIAN_POINT ( 'NONE',  ( -30.00000000000002842, -225.0000000000000000, 190.0000000000000000 ) ) ;
#12633=EDGE_CURVE ( 'NONE', #13795, #4174, #9678, .T. ) ;
#12634=DIRECTION ( 'NONE',  ( 0.000000000000000000, 0.000000000000000000, -1.000000000000000000 ) ) ;
#12640=CYLINDRICAL_SURFACE ( 'NONE', #10630, 5.500000000000005329 ) ;
#12646=ORIENTED_EDGE ( 'NONE', *, *, #12785, .T. ) ;
#12653=AXIS2_PLACEMENT_3D ( 'NONE', #5655, #10079, #13476 ) ;
#12654=ORIENTED_EDGE ( 'NONE', *, *, #2992, .T. ) ;
#12659=ADVANCED_FACE ( 'NONE', ( #1370 ), #7039, .F. ) ;
#12664=AXIS2_PLACEMENT_3D ( 'NONE', #6187, #8360, #3869 ) ;
#12666=DIRECTION ( 'NONE',  ( -1.000000000000000000, 0.000000000000000000, 0.000000000000000000 ) ) ;
#12671=ORIENTED_EDGE ( 'NONE', *, *, #3848, .T. ) ;
#12673=ADVANCED_FACE ( 'NONE', ( #11467 ), #12480, .F. ) ;
#12676=AXIS2_PLACEMENT_3D ( 'NONE', #65, #4525, #207 ) ;
#12688=CYLINDRICAL_SURFACE ( 'NONE', #10042, 2.649999999999985700 ) ;
#12689=DIRECTION ( 'NONE',  ( 1.000000000000000000, 0.000000000000000000, 0.000000000000000000 ) ) ;
#12698=LINE ( 'NONE', #2768, #13835 ) ;
#12699=CARTESIAN_POINT ( 'NONE',  ( 470.0000000000000000, -25.00000000000000000, 250.0000000000000000 ) ) ;
#12700=DIRECTION ( 'NONE',  ( 0.000000000000000000, 0.000000000000000000, -1.000000000000000000 ) ) ;
#12706=EDGE_CURVE ( 'NONE', #11791, #5335, #2016, .T. ) ;
#12707=ORIENTED_EDGE ( 'NONE', *, *, #5092, .F. ) ;
#12709=ADVANCED_FACE ( 'NONE', ( #11398 ), #13704, .T. ) ;
#12714=ORIENTED_EDGE ( 'NONE', *, *, #5774, .T. ) ;
#12716=ADVANCED_FACE ( 'NONE', ( #3566, #4874 ), #10299, .F. ) ;
#12719=LINE ( 'NONE', #7989, #12017 ) ;
#12720=CARTESIAN_POINT ( 'NONE',  ( 136.6666666666666288, -20.00000000000000000, -219.8500000000001080 ) ) ;
#12725=ORIENTED_EDGE ( 'NONE', *, *, #9241, .F. ) ;
#12730=CARTESIAN_POINT ( 'NONE',  ( -30.00000000000002842, -225.0000000000000000, 169.9999999999999716 ) ) ;
#12739=CARTESIAN_POINT ( 'NONE',  ( 302.6499999999999204, -95.00000000000008527, -190.0000000000000000 ) ) ;
#12746=CARTESIAN_POINT ( 'NONE',  ( 119.9999999999999147, -20.00000000000000000, 169.9999999999999716 ) ) ;
#12747=EDGE_CURVE ( 'NONE', #4602, #13282, #6662, .T. ) ;
#12748=AXIS2_PLACEMENT_3D ( 'NONE', #3822, #7020, #8234 ) ;
#12759=EDGE_CURVE ( 'NONE', #10523, #5871, #4798, .T. ) ;
#12761=ORIENTED_EDGE ( 'NONE', *, *, #1602, .T. ) ;
#12768=AXIS2_PLACEMENT_3D ( 'NONE', #6485, #10772, #8512 ) ;
#12770=DIRECTION ( 'NONE',  ( -0.000000000000000000, -0.000000000000000000, 1.000000000000000000 ) ) ;
#12771=VERTEX_POINT ( 'NONE', #2623 ) ;
#12777=CYLINDRICAL_SURFACE ( 'NONE', #12288, 2.500000000000002220 ) ;
#12781=ORIENTED_EDGE ( 'NONE', *, *, #3434, .F. ) ;
#12785=EDGE_CURVE ( 'NONE', #9136, #6389, #9912, .T. ) ;
#12790=ORIENTED_EDGE ( 'NONE', *, *, #2022, .F. ) ;
#12791=DIRECTION ( 'NONE',  ( 0.000000000000000000, 0.000000000000000000, 1.000000000000000000 ) ) ;
#12792=ORIENTED_EDGE ( 'NONE', *, *, #3399, .T. ) ;
#12793=LINE ( 'NONE', #10471, #1295 ) ;
#12801=CARTESIAN_POINT ( 'NONE',  ( 305.4999999999999432, -75.00000000000008527, -190.0000000000000000 ) ) ;
#12815=CARTESIAN_POINT ( 'NONE',  ( 134.5000000000000000, -95.00000000000008527, 190.0000000000000000 ) ) ;
#12816=DIRECTION ( 'NONE',  ( -0.000000000000000000, -0.000000000000000000, 1.000000000000000000 ) ) ;
#12822=DIRECTION ( 'NONE',  ( 0.000000000000000000, 0.000000000000000000, -1.000000000000000000 ) ) ;
#12825=DIRECTION ( 'NONE',  ( 0.000000000000000000, 0.000000000000000000, -1.000000000000000000 ) ) ;
#12831=PLANE ( 'NONE',  #7760 ) ;
#12836=CARTESIAN_POINT ( 'NONE',  ( 137.4999999999999432, -36.99999999999997868, -169.9999999999999716 ) ) ;
#12845=ADVANCED_BREP_SHAPE_REPRESENTATION ( '', ( #3574, #14039 ), #7000 ) ;
#12846=CARTESIAN_POINT ( 'NONE',  ( 142.6500000000000057, -75.00000000000008527, 186.2999999999999829 ) ) ;
#12847=VERTEX_POINT ( 'NONE', #8263 ) ;
#12858=DIRECTION ( 'NONE',  ( 0.000000000000000000, 0.000000000000000000, -1.000000000000000000 ) ) ;
#12859=EDGE_CURVE ( 'NONE', #5386, #10300, #13147, .T. ) ;
#12867=EDGE_CURVE ( 'NONE', #12771, #9739, #9584, .T. ) ;
#12869=AXIS2_PLACEMENT_3D ( 'NONE', #7700, #14228, #11854 ) ;
#12874=CARTESIAN_POINT ( 'NONE',  ( 140.0000000000000000, -95.00000000000008527, 169.9999999999999716 ) ) ;
#12878=CIRCLE ( 'NONE', #2449, 2.500000000000002220 ) ;
#12879=DIRECTION ( 'NONE',  ( -0.000000000000000000, -0.000000000000000000, 1.000000000000000000 ) ) ;
#12884=VERTEX_POINT ( 'NONE', #12836 ) ;
#12890=AXIS2_PLACEMENT_3D ( 'NONE', #11560, #8431, #10627 ) ;
#12892=FACE_OUTER_BOUND ( 'NONE', #4329, .T. ) ;
#12895=DIRECTION ( 'NONE',  ( -0.000000000000000000, -0.000000000000000000, 1.000000000000000000 ) ) ;
#12898=VECTOR ( 'NONE', #9279, 1000.000000000000000 ) ;
#12899=DIRECTION ( 'NONE',  ( -0.000000000000000000, -0.000000000000000000, -1.000000000000000000 ) ) ;
#12902=VERTEX_POINT ( 'NONE', #7320 ) ;
#12903=AXIS2_PLACEMENT_3D ( 'NONE', #8579, #6404, #6185 ) ;
#12904=FACE_OUTER_BOUND ( 'NONE', #7490, .T. ) ;
#12906=ORIENTED_EDGE ( 'NONE', *, *, #12094, .T. ) ;
#12907=PLANE ( 'NONE',  #9343 ) ;
#12908=DIRECTION ( 'NONE',  ( -0.000000000000000000, -0.000000000000000000, 1.000000000000000000 ) ) ;
#12912=ORIENTED_EDGE ( 'NONE', *, *, #13545, .T. ) ;
#12913=CARTESIAN_POINT ( 'NONE',  ( 294.4999999999999432, -95.00000000000008527, -190.0000000000000000 ) ) ;
#12920=VECTOR ( 'NONE', #12770, 1000.000000000000000 ) ;
#12923=FACE_OUTER_BOUND ( 'NONE', #3347, .T. ) ;
#12930=EDGE_LOOP ( 'NONE', ( #6652, #6583, #738, #7282 ) ) ;
#12936=LINE ( 'NONE', #14012, #365 ) ;
#12943=EDGE_LOOP ( 'NONE', ( #9068, #1176, #10591, #715, #5602, #11444, #6251, #3095, #10440, #3890, #7728, #13420 ) ) ;
#12949=ORIENTED_EDGE ( 'NONE', *, *, #12706, .T. ) ;
#12950=AXIS2_PLACEMENT_3D ( 'NONE', #2675, #13694, #3770 ) ;
#12957=ORIENTED_EDGE ( 'NONE', *, *, #4791, .T. ) ;
#12959=AXIS2_PLACEMENT_3D ( 'NONE', #1795, #6228, #13980 ) ;
#12969=DIRECTION ( 'NONE',  ( -0.000000000000000000, -0.000000000000000000, -1.000000000000000000 ) ) ;
#12970=VECTOR ( 'NONE', #13091, 1000.000000000000000 ) ;
#12971=EDGE_CURVE ( 'NONE', #9959, #1020, #6721, .T. ) ;
#12977=EDGE_CURVE ( 'NONE', #9413, #5437, #11296, .T. ) ;
#12981=CARTESIAN_POINT ( 'NONE',  ( 299.9999999999999432, -95.00000000000008527, 186.2999999999999829 ) ) ;
#12982=EDGE_LOOP ( 'NONE', ( #3805, #10349, #4978, #7812 ) ) ;
#12987=EDGE_LOOP ( 'NONE', ( #8122, #4214, #5308, #2385 ) ) ;
#12989=ORIENTED_EDGE ( 'NONE', *, *, #12759, .F. ) ;
#12995=DIRECTION ( 'NONE',  ( -0.000000000000000000, -1.000000000000000000, -0.000000000000000000 ) ) ;
#13009=ORIENTED_EDGE ( 'NONE', *, *, #3061, .T. ) ;
#13017=AXIS2_PLACEMENT_3D ( 'NONE', #11708, #5121, #2179 ) ;
#13019=DIRECTION ( 'NONE',  ( -0.000000000000000000, 1.000000000000000000, -0.000000000000000000 ) ) ;
#13023=ORIENTED_EDGE ( 'NONE', *, *, #12358, .F. ) ;
#13026=EDGE_CURVE ( 'NONE', #4429, #12042, #13520, .T. ) ;
#13028=CYLINDRICAL_SURFACE ( 'NONE', #4176, 2.649999999999985700 ) ;
#13035=AXIS2_PLACEMENT_3D ( 'NONE', #9830, #14238, #1578 ) ;
#13042=EDGE_CURVE ( 'NONE', #2872, #10967, #5698, .T. ) ;
#13050=ORIENTED_EDGE ( 'NONE', *, *, #11691, .F. ) ;
#13055=ORIENTED_EDGE ( 'NONE', *, *, #11917, .T. ) ;
#13066=ORIENTED_EDGE ( 'NONE', *, *, #11011, .T. ) ;
#13075=CARTESIAN_POINT ( 'NONE',  ( 134.5000000000000000, -75.00000000000008527, -190.0000000000000000 ) ) ;
#13076=CARTESIAN_POINT ( 'NONE',  ( 238.9999999999999432, -85.00000000000007105, 180.0000000000000000 ) ) ;
#13088=FACE_OUTER_BOUND ( 'NONE', #1672, .T. ) ;
#13090=CYLINDRICAL_SURFACE ( 'NONE', #2817, 5.500000000000005329 ) ;
#13091=DIRECTION ( 'NONE',  ( 0.8571673013836870192, 0.000000000000000000, 0.5150380737757234151 ) ) ;
#13096=ORIENTED_EDGE ( 'NONE', *, *, #3563, .F. ) ;
#13101=FACE_OUTER_BOUND ( 'NONE', #10010, .T. ) ;
#13108=CIRCLE ( 'NONE', #2937, 5.500000000000005329 ) ;
#13125=AXIS2_PLACEMENT_3D ( 'NONE', #9036, #7800, #7939 ) ;
#13132=CIRCLE ( 'NONE', #11997, 2.649999999999985700 ) ;
#13143=ORIENTED_EDGE ( 'NONE', *, *, #5037, .F. ) ;
#13147=CIRCLE ( 'NONE', #12225, 2.649999999999985700 ) ;
#13151=DIRECTION ( 'NONE',  ( 1.000000000000000000, 0.000000000000000000, 0.000000000000000000 ) ) ;
#13152=CIRCLE ( 'NONE', #10614, 5.500000000000005329 ) ;
#13160=ORIENTED_EDGE ( 'NONE', *, *, #12353, .T. ) ;
#13161=EDGE_CURVE ( 'NONE', #14007, #11339, #626, .T. ) ;
#13177=DIRECTION ( 'NONE',  ( -0.000000000000000000, -0.000000000000000000, 1.000000000000000000 ) ) ;
#13180=EDGE_CURVE ( 'NONE', #9652, #13843, #3811, .T. ) ;
#13183=DIRECTION ( 'NONE',  ( -0.000000000000000000, -0.000000000000000000, -1.000000000000000000 ) ) ;
#13186=VECTOR ( 'NONE', #2161, 1000.000000000000000 ) ;
#13187=EDGE_LOOP ( 'NONE', ( #7692, #2042 ) ) ;
#13192=EDGE_CURVE ( 'NONE', #7698, #10043, #12009, .T. ) ;
#13200=CARTESIAN_POINT ( 'NONE',  ( -30.00000000000002842, -225.0000000000000000, -190.0000000000000000 ) ) ;
#13203=CARTESIAN_POINT ( 'NONE',  ( 305.0000000000000000, -36.99999999999997868, -169.9999999999999716 ) ) ;
#13205=ADVANCED_FACE ( 'NONE', ( #4319, #11942, #6354, #7290, #9834, #9698, #9548, #6275, #5341 ), #4255, .T. ) ;
#13214=VECTOR ( 'NONE', #13177, 1000.000000000000000 ) ;
#13231=ORIENTED_EDGE ( 'NONE', *, *, #4827, .T. ) ;
#13233=ORIENTED_EDGE ( 'NONE', *, *, #9700, .T. ) ;
#13240=ADVANCED_FACE ( 'NONE', ( #8670, #3024, #7438, #11869, #6207, #812, #8742, #13088 ), #3170, .T. ) ;
#13243=EDGE_CURVE ( 'NONE', #7848, #2165, #6209, .T. ) ;
#13249=FACE_OUTER_BOUND ( 'NONE', #4029, .T. ) ;
#13250=LINE ( 'NONE', #6794, #1866 ) ;
#13251=CIRCLE ( 'NONE', #8378, 2.500000000000002220 ) ;
#13253=ORIENTED_EDGE ( 'NONE', *, *, #6736, .F. ) ;
#13257=FACE_OUTER_BOUND ( 'NONE', #12987, .T. ) ;
#13261=EDGE_CURVE ( 'NONE', #328, #8099, #7507, .T. ) ;
#13264=AXIS2_PLACEMENT_3D ( 'NONE', #10639, #11721, #5275 ) ;
#13266=DIRECTION ( 'NONE',  ( 1.000000000000000000, 0.000000000000000000, 0.000000000000000000 ) ) ;
#13268=ORIENTED_EDGE ( 'NONE', *, *, #266, .T. ) ;
#13270=CARTESIAN_POINT ( 'NONE',  ( 233.9999999999999432, -85.00000000000007105, 180.0000000000000000 ) ) ;
#13274=VERTEX_POINT ( 'NONE', #181 ) ;
#13279=ORIENTED_EDGE ( 'NONE', *, *, #7895, .T. ) ;
#13280=VERTEX_POINT ( 'NONE', #13440 ) ;
#13282=VERTEX_POINT ( 'NONE', #6846 ) ;
#13299=EDGE_CURVE ( 'NONE', #4498, #13983, #9981, .T. ) ;
#13302=DIRECTION ( 'NONE',  ( -0.000000000000000000, -0.000000000000000000, -1.000000000000000000 ) ) ;
#13303=ORIENTED_EDGE ( 'NONE', *, *, #12241, .F. ) ;
#13311=ORIENTED_EDGE ( 'NONE', *, *, #3219, .F. ) ;
#13319=CARTESIAN_POINT ( 'NONE',  ( -30.00000000000002842, -25.00000000000000000, 190.0000000000000000 ) ) ;
#13322=EDGE_CURVE ( 'NONE', #1452, #12590, #1801, .T. ) ;
#13325=CARTESIAN_POINT ( 'NONE',  ( 145.5000000000000284, -75.00000000000008527, 190.0000000000000000 ) ) ;
#13334=CARTESIAN_POINT ( 'NONE',  ( 119.9999999999999147, -225.0010000000000048, 19.99999999999998934 ) ) ;
#13340=AXIS2_PLACEMENT_3D ( 'NONE', #5883, #3783, #331 ) ;
#13342=ORIENTED_EDGE ( 'NONE', *, *, #9106, .T. ) ;
#13346=AXIS2_PLACEMENT_3D ( 'NONE', #8567, #11040, #8857 ) ;
#13350=CARTESIAN_POINT ( 'NONE',  ( 386.6666666666666288, -20.00000000000000000, -222.5000000000000853 ) ) ;
#13354=EDGE_CURVE ( 'NONE', #4498, #3293, #6449, .T. ) ;
#13367=CARTESIAN_POINT ( 'NONE',  ( 319.9999999999999432, -20.00000000000000000, 169.9999999999999716 ) ) ;
#13379=EDGE_CURVE ( 'NONE', #9474, #2746, #2207, .T. ) ;
#13382=AXIS2_PLACEMENT_3D ( 'NONE', #2357, #3244, #7854 ) ;
#13384=ORIENTED_EDGE ( 'NONE', *, *, #13261, .F. ) ;
#13396=DIRECTION ( 'NONE',  ( 1.000000000000000000, 0.000000000000000000, 0.000000000000000000 ) ) ;
#13398=ORIENTED_EDGE ( 'NONE', *, *, #665, .T. ) ;
#13402=FACE_OUTER_BOUND ( 'NONE', #7371, .T. ) ;
#13406=LINE ( 'NONE', #7955, #11627 ) ;
#13413=ORIENTED_EDGE ( 'NONE', *, *, #7963, .F. ) ;
#13417=AXIS2_PLACEMENT_3D ( 'NONE', #14107, #12879, #523 ) ;
#13420=ORIENTED_EDGE ( 'NONE', *, *, #2616, .T. ) ;
#13423=LINE ( 'NONE', #10985, #14287 ) ;
#13424=CARTESIAN_POINT ( 'NONE',  ( 219.9999999999999716, -25.00000000000000000, 225.1500000000000625 ) ) ;
#13428=FACE_BOUND ( 'NONE', #4170, .T. ) ;
#13434=ORIENTED_EDGE ( 'NONE', *, *, #10798, .T. ) ;
#13435=EDGE_CURVE ( 'NONE', #634, #5319, #11487, .T. ) ;
#13440=CARTESIAN_POINT ( 'NONE',  ( 136.6666666666666288, -25.00000000000000000, 219.8500000000001080 ) ) ;
#13449=EDGE_CURVE ( 'NONE', #10366, #10615, #8140, .T. ) ;
#13453=DIRECTION ( 'NONE',  ( 0.8571673013836870192, 0.000000000000000000, 0.5150380737757234151 ) ) ;
#13466=EDGE_LOOP ( 'NONE', ( #1499, #7573, #8252, #3239 ) ) ;
#13476=DIRECTION ( 'NONE',  ( 1.000000000000000000, 0.000000000000000000, 0.000000000000000000 ) ) ;
#13482=ORIENTED_EDGE ( 'NONE', *, *, #1252, .F. ) ;
#13486=ADVANCED_FACE ( 'NONE', ( #10397 ), #12640, .F. ) ;
#13491=PLANE ( 'NONE',  #7704 ) ;
#13501=DIRECTION ( 'NONE',  ( -0.000000000000000000, -0.000000000000000000, 1.000000000000000000 ) ) ;
#13504=EDGE_CURVE ( 'NONE', #13543, #12061, #12719, .T. ) ;
#13506=DIRECTION ( 'NONE',  ( 1.000000000000000000, 0.000000000000000000, 0.000000000000000000 ) ) ;
#13512=CARTESIAN_POINT ( 'NONE',  ( 469.9999999999998863, -225.0000000000000000, 169.9999999999999716 ) ) ;
#13514=DIRECTION ( 'NONE',  ( 1.000000000000000000, 0.000000000000000000, 0.000000000000000000 ) ) ;
#13518=CARTESIAN_POINT ( 'NONE',  ( 299.9999999999999432, -95.00000000000008527, 190.0000000000000000 ) ) ;
#13520=LINE ( 'NONE', #9111, #10608 ) ;
#13524=CARTESIAN_POINT ( 'NONE',  ( 219.9999999999999716, -20.00000000000000000, -225.1500000000000625 ) ) ;
#13526=ORIENTED_EDGE ( 'NONE', *, *, #12338, .F. ) ;
#13530=ORIENTED_EDGE ( 'NONE', *, *, #5626, .T. ) ;
#13531=VERTEX_POINT ( 'NONE', #13076 ) ;
#13532=PLANE ( 'NONE',  #13562 ) ;
#13538=CYLINDRICAL_SURFACE ( 'NONE', #3525, 2.649999999999985700 ) ;
#13539=CARTESIAN_POINT ( 'NONE',  ( 145.5000000000000284, -95.00000000000008527, 186.2999999999999829 ) ) ;
#13543=VERTEX_POINT ( 'NONE', #3159 ) ;
#13544=ORIENTED_EDGE ( 'NONE', *, *, #4743, .F. ) ;
#13545=EDGE_CURVE ( 'NONE', #13274, #10393, #7597, .T. ) ;
#13546=LINE ( 'NONE', #192, #6374 ) ;
#13552=VERTEX_POINT ( 'NONE', #7346 ) ;
#13553=DIRECTION ( 'NONE',  ( 0.000000000000000000, 0.000000000000000000, 1.000000000000000000 ) ) ;
#13562=AXIS2_PLACEMENT_3D ( 'NONE', #2603, #8237, #4715 ) ;
#13569=ORIENTED_EDGE ( 'NONE', *, *, #1056, .F. ) ;
#13571=VERTEX_POINT ( 'NONE', #3948 ) ;
#13580=EDGE_CURVE ( 'NONE', #13983, #3594, #4112, .T. ) ;
#13590=EDGE_CURVE ( 'NONE', #2924, #7600, #12936, .T. ) ;
#13596=DIRECTION ( 'NONE',  ( 1.000000000000000000, 0.000000000000000000, 0.000000000000000000 ) ) ;
#13603=DIRECTION ( 'NONE',  ( 0.000000000000000000, 0.000000000000000000, -1.000000000000000000 ) ) ;
#13605=DIRECTION ( 'NONE',  ( 0.000000000000000000, 0.000000000000000000, -1.000000000000000000 ) ) ;
#13608=CARTESIAN_POINT ( 'NONE',  ( 140.0000000000000000, -95.00000000000008527, 186.2999999999999829 ) ) ;
#13611=ORIENTED_EDGE ( 'NONE', *, *, #2022, .T. ) ;
#13613=FACE_BOUND ( 'NONE', #10198, .T. ) ;
#13616=DIRECTION ( 'NONE',  ( 0.000000000000000000, -0.000000000000000000, -1.000000000000000000 ) ) ;
#13619=AXIS2_PLACEMENT_3D ( 'NONE', #6851, #12299, #5688 ) ;
#13626=ORIENTED_EDGE ( 'NONE', *, *, #9596, .T. ) ;
#13627=CARTESIAN_POINT ( 'NONE',  ( 386.6666666666666288, -25.00000000000000000, 222.5000000000000853 ) ) ;
#13640=DIRECTION ( 'NONE',  ( 1.000000000000000000, 0.000000000000000000, 0.000000000000000000 ) ) ;
#13642=CARTESIAN_POINT ( 'NONE',  ( 299.9999999999999432, -75.00000000000008527, 186.2999999999999829 ) ) ;
#13643=ORIENTED_EDGE ( 'NONE', *, *, #9018, .T. ) ;
#13647=CARTESIAN_POINT ( 'NONE',  ( 219.9999999999999716, -85.00000000000007105, 190.0000000000000000 ) ) ;
#13650=DIRECTION ( 'NONE',  ( -0.000000000000000000, -0.000000000000000000, 1.000000000000000000 ) ) ;
#13651=VERTEX_POINT ( 'NONE', #8658 ) ;
#13655=VECTOR ( 'NONE', #13736, 1000.000000000000000 ) ;
#13656=EDGE_CURVE ( 'NONE', #9120, #9740, #5328, .T. ) ;
#13658=DIRECTION ( 'NONE',  ( 1.000000000000000000, 0.000000000000000000, 0.000000000000000000 ) ) ;
#13661=( LENGTH_UNIT ( ) NAMED_UNIT ( * ) SI_UNIT ( .MILLI., .METRE. ) );
#13669=AXIS2_PLACEMENT_3D ( 'NONE', #8828, #12155, #13506 ) ;
#13671=CARTESIAN_POINT ( 'NONE',  ( 132.4999999999999432, -56.99999999999997158, -169.9999999999999716 ) ) ;
#13674=ORIENTED_EDGE ( 'NONE', *, *, #2672, .F. ) ;
#13675=CIRCLE ( 'NONE', #7873, 2.649999999999985700 ) ;
#13686=ORIENTED_EDGE ( 'NONE', *, *, #9415, .F. ) ;
#13687=DIRECTION ( 'NONE',  ( -0.000000000000000000, -0.000000000000000000, -1.000000000000000000 ) ) ;
#13694=DIRECTION ( 'NONE',  ( -0.000000000000000000, -0.000000000000000000, 1.000000000000000000 ) ) ;
#13697=VERTEX_POINT ( 'NONE', #7904 ) ;
#13702=CARTESIAN_POINT ( 'NONE',  ( 140.0000000000000000, -95.00000000000008527, 169.9999999999999716 ) ) ;
#13704=PLANE ( 'NONE',  #11996 ) ;
#13713=COLOUR_RGB ( '',0.8941176470588234615, 0.8941176470588234615, 0.8941176470588234615 ) ;
#13717=DIRECTION ( 'NONE',  ( 0.000000000000000000, 0.000000000000000000, -1.000000000000000000 ) ) ;
#13721=AXIS2_PLACEMENT_3D ( 'NONE', #8814, #11071, #9833 ) ;
#13722=ORIENTED_EDGE ( 'NONE', *, *, #234, .F. ) ;
#13723=LINE ( 'NONE', #4818, #1152 ) ;
#13727=ORIENTED_EDGE ( 'NONE', *, *, #9735, .T. ) ;
#13729=ORIENTED_EDGE ( 'NONE', *, *, #14217, .T. ) ;
#13736=DIRECTION ( 'NONE',  ( 0.000000000000000000, 0.000000000000000000, -1.000000000000000000 ) ) ;
#13743=FACE_OUTER_BOUND ( 'NONE', #2111, .T. ) ;
#13752=ORIENTED_EDGE ( 'NONE', *, *, #530, .F. ) ;
#13753=EDGE_CURVE ( 'NONE', #7324, #5335, #13423, .T. ) ;
#13760=ADVANCED_FACE ( 'NONE', ( #10094 ), #3297, .F. ) ;
#13763=CARTESIAN_POINT ( 'NONE',  ( -30.00000000000002842, -25.00000000000000000, 250.0000000000000000 ) ) ;
#13768=EDGE_LOOP ( 'NONE', ( #5699, #3083, #13434, #13686 ) ) ;
#13769=ADVANCED_FACE ( 'NONE', ( #3370 ), #4590, .F. ) ;
#13770=DIRECTION ( 'NONE',  ( 1.000000000000000000, 0.000000000000000000, -0.000000000000000000 ) ) ;
#13773=CARTESIAN_POINT ( 'NONE',  ( 145.5000000000000284, -75.00000000000008527, 190.0000000000000000 ) ) ;
#13778=DIRECTION ( 'NONE',  ( -0.000000000000000000, -0.000000000000000000, -1.000000000000000000 ) ) ;
#13780=ORIENTED_EDGE ( 'NONE', *, *, #5091, .T. ) ;
#13795=VERTEX_POINT ( 'NONE', #7767 ) ;
#13803=AXIS2_PLACEMENT_3D ( 'NONE', #13203, #1141, #186 ) ;
#13806=AXIS2_PLACEMENT_3D ( 'NONE', #10146, #2312, #6553 ) ;
#13807=VECTOR ( 'NONE', #10922, 1000.000000000000000 ) ;
#13810=VECTOR ( 'NONE', #3488, 1000.000000000000000 ) ;
#13811=ORIENTED_EDGE ( 'NONE', *, *, #5803, .T. ) ;
#13828=FACE_OUTER_BOUND ( 'NONE', #11167, .T. ) ;
#13831=FACE_OUTER_BOUND ( 'NONE', #7867, .T. ) ;
#13833=DIRECTION ( 'NONE',  ( 0.000000000000000000, 0.000000000000000000, 1.000000000000000000 ) ) ;
#13835=VECTOR ( 'NONE', #5020, 1000.000000000000000 ) ;
#13843=VERTEX_POINT ( 'NONE', #2627 ) ;
#13846=EDGE_CURVE ( 'NONE', #3377, #12061, #10303, .T. ) ;
#13849=EDGE_CURVE ( 'NONE', #6716, #11552, #2018, .T. ) ;
#13853=FACE_OUTER_BOUND ( 'NONE', #2144, .T. ) ;
#13865=ORIENTED_EDGE ( 'NONE', *, *, #11621, .F. ) ;
#13866=DIRECTION ( 'NONE',  ( 0.000000000000000000, 0.000000000000000000, 1.000000000000000000 ) ) ;
#13869=DIRECTION ( 'NONE',  ( -1.000000000000000000, 0.000000000000000000, 0.000000000000000000 ) ) ;
#13872=DIRECTION ( 'NONE',  ( -0.000000000000000000, -0.000000000000000000, -1.000000000000000000 ) ) ;
#13873=DIRECTION ( 'NONE',  ( -0.000000000000000000, -0.000000000000000000, -1.000000000000000000 ) ) ;
#13876=AXIS2_PLACEMENT_3D ( 'NONE', #9789, #7737, #8688 ) ;
#13887=ORIENTED_EDGE ( 'NONE', *, *, #1415, .F. ) ;
#13888=CIRCLE ( 'NONE', #10416, 2.649999999999985700 ) ;
#13899=EDGE_CURVE ( 'NONE', #11802, #9015, #13132, .T. ) ;
#13900=EDGE_LOOP ( 'NONE', ( #14131, #1389 ) ) ;
#13905=DIRECTION ( 'NONE',  ( 0.000000000000000000, 1.000000000000000000, 0.000000000000000000 ) ) ;
#13906=CARTESIAN_POINT ( 'NONE',  ( 319.9999999999999432, -24.99999999999999289, 19.99999999999998934 ) ) ;
#13922=CARTESIAN_POINT ( 'NONE',  ( 299.9999999999999432, -95.00000000000008527, 186.2999999999999829 ) ) ;
#13926=DIRECTION ( 'NONE',  ( 0.000000000000000000, 0.000000000000000000, -1.000000000000000000 ) ) ;
#13938=EDGE_LOOP ( 'NONE', ( #8886, #1734 ) ) ;
#13940=CIRCLE ( 'NONE', #13017, 2.500000000000002220 ) ;
#13943=VERTEX_POINT ( 'NONE', #6970 ) ;
#13948=CYLINDRICAL_SURFACE ( 'NONE', #1418, 2.649999999999985700 ) ;
#13950=EDGE_CURVE ( 'NONE', #1808, #9732, #4339, .T. ) ;
#13951=CARTESIAN_POINT ( 'NONE',  ( 53.33333333333330017, -20.00000000000000000, -219.8500000000001080 ) ) ;
#13953=EDGE_CURVE ( 'NONE', #7861, #6913, #601, .T. ) ;
#13958=CIRCLE ( 'NONE', #5402, 2.649999999999985700 ) ;
#13964=AXIS2_PLACEMENT_3D ( 'NONE', #6271, #5054, #14167 ) ;
#13965=DIRECTION ( 'NONE',  ( 1.000000000000000000, 0.000000000000000000, 0.000000000000000000 ) ) ;
#13967=SURFACE_STYLE_USAGE ( .BOTH. , #11058 ) ;
#13977=DIRECTION ( 'NONE',  ( -0.000000000000000000, -0.000000000000000000, -1.000000000000000000 ) ) ;
#13980=DIRECTION ( 'NONE',  ( 0.000000000000000000, 0.000000000000000000, 1.000000000000000000 ) ) ;
#13983=VERTEX_POINT ( 'NONE', #201 ) ;
#13984=FACE_BOUND ( 'NONE', #5111, .T. ) ;
#13987=LINE ( 'NONE', #12616, #1668 ) ;
#13991=DIRECTION ( 'NONE',  ( -0.000000000000000000, -0.000000000000000000, -1.000000000000000000 ) ) ;
#13994=EDGE_LOOP ( 'NONE', ( #12949, #8264 ) ) ;
#13995=DIRECTION ( 'NONE',  ( 0.000000000000000000, 0.000000000000000000, -1.000000000000000000 ) ) ;
#14007=VERTEX_POINT ( 'NONE', #14070 ) ;
#14009=EDGE_LOOP ( 'NONE', ( #10254, #9706 ) ) ;
#14012=CARTESIAN_POINT ( 'NONE',  ( -30.00000000000002842, -225.0000000000000000, -169.9999999999999716 ) ) ;
#14013=DIRECTION ( 'NONE',  ( -0.000000000000000000, 0.000000000000000000, 1.000000000000000000 ) ) ;
#14015=FACE_OUTER_BOUND ( 'NONE', #10138, .T. ) ;
#14018=CARTESIAN_POINT ( 'NONE',  ( 142.6500000000000057, -95.00000000000008527, 186.2999999999999829 ) ) ;
#14019=ORIENTED_EDGE ( 'NONE', *, *, #326, .F. ) ;
#14034=EDGE_CURVE ( 'NONE', #12590, #5504, #8339, .T. ) ;
#14035=VECTOR ( 'NONE', #13778, 1000.000000000000000 ) ;
#14038=DIRECTION ( 'NONE',  ( -1.000000000000000000, 0.000000000000000000, 0.000000000000000000 ) ) ;
#14039=AXIS2_PLACEMENT_3D ( 'NONE', #10508, #9418, #5077 ) ;
#14042=LINE ( 'NONE', #9844, #14130 ) ;
#14044=DIRECTION ( 'NONE',  ( -0.000000000000000000, -1.000000000000000000, -0.000000000000000000 ) ) ;
#14046=PRODUCT_DEFINITION_CONTEXT ( 'detailed design', #5364, 'design' ) ;
#14052=CARTESIAN_POINT ( 'NONE',  ( 219.9999999999999716, -20.00000000000000000, 222.5000000000000853 ) ) ;
#14058=CIRCLE ( 'NONE', #4576, 2.500000000000002220 ) ;
#14059=DIRECTION ( 'NONE',  ( 0.000000000000000000, 0.000000000000000000, 1.000000000000000000 ) ) ;
#14064=AXIS2_PLACEMENT_3D ( 'NONE', #13642, #11201, #1522 ) ;
#14066=DIRECTION ( 'NONE',  ( -0.000000000000000000, 0.000000000000000000, 1.000000000000000000 ) ) ;
#14069=AXIS2_PLACEMENT_3D ( 'NONE', #7884, #7750, #3483 ) ;
#14070=CARTESIAN_POINT ( 'NONE',  ( 303.3333333333333144, -25.00000000000000000, -225.1500000000000625 ) ) ;
#14072=DIRECTION ( 'NONE',  ( 1.000000000000000000, 0.000000000000000000, 0.000000000000000000 ) ) ;
#14077=DIRECTION ( 'NONE',  ( 1.000000000000000000, 0.000000000000000000, 0.000000000000000000 ) ) ;
#14078=EDGE_CURVE ( 'NONE', #4429, #12208, #7085, .T. ) ;
#14085=UNCERTAINTY_MEASURE_WITH_UNIT (LENGTH_MEASURE( 1.000000000000000082E-05 ), #5987, 'distance_accuracy_value', 'NONE');
#14087=AXIS2_PLACEMENT_3D ( 'NONE', #2423, #7782, #8815 ) ;
#14092=FACE_OUTER_BOUND ( 'NONE', #6253, .T. ) ;
#14094=DIRECTION ( 'NONE',  ( 1.000000000000000000, 0.000000000000000000, 0.000000000000000000 ) ) ;
#14095=DIRECTION ( 'NONE',  ( -0.000000000000000000, -0.000000000000000000, -1.000000000000000000 ) ) ;
#14100=EDGE_LOOP ( 'NONE', ( #5109, #13160 ) ) ;
#14104=ORIENTED_EDGE ( 'NONE', *, *, #9865, .T. ) ;
#14107=CARTESIAN_POINT ( 'NONE',  ( 299.9999999999999432, -95.00000000000008527, 169.9999999999999716 ) ) ;
#14113=EDGE_CURVE ( 'NONE', #840, #1382, #11044, .T. ) ;
#14119=CARTESIAN_POINT ( 'NONE',  ( 297.3499999999999659, -95.00000000000008527, -169.9999999999999716 ) ) ;
#14123=AXIS2_PLACEMENT_3D ( 'NONE', #10681, #9448, #712 ) ;
#14129=CIRCLE ( 'NONE', #7185, 2.500000000000002220 ) ;
#14130=VECTOR ( 'NONE', #8680, 1000.000000000000000 ) ;
#14131=ORIENTED_EDGE ( 'NONE', *, *, #5577, .T. ) ;
#14134=CARTESIAN_POINT ( 'NONE',  ( 297.3499999999999659, -75.00000000000008527, -169.9999999999999716 ) ) ;
#14137=FACE_BOUND ( 'NONE', #5955, .T. ) ;
#14138=ADVANCED_FACE ( 'NONE', ( #13402 ), #2176, .T. ) ;
#14142=CARTESIAN_POINT ( 'NONE',  ( 134.9999999999999432, -56.99999999999997158, -169.9999999999999716 ) ) ;
#14148=PLANE ( 'NONE',  #3135 ) ;
#14150=( GEOMETRIC_REPRESENTATION_CONTEXT ( 3 ) GLOBAL_UNCERTAINTY_ASSIGNED_CONTEXT ( ( #4021 ) ) GLOBAL_UNIT_ASSIGNED_CONTEXT ( ( #13661, #5123, #9541 ) ) REPRESENTATION_CONTEXT ( 'NONE', 'WORKASPACE' ) );
#14151=CARTESIAN_POINT ( 'NONE',  ( 319.9999999999999432, -225.0010000000000048, 19.99999999999998934 ) ) ;
#14153=EDGE_LOOP ( 'NONE', ( #12551, #9627, #13096, #9429 ) ) ;
#14154=CARTESIAN_POINT ( 'NONE',  ( 140.0000000000000000, -75.00000000000008527, 186.2999999999999829 ) ) ;
#14162=ORIENTED_EDGE ( 'NONE', *, *, #12977, .F. ) ;
#14167=DIRECTION ( 'NONE',  ( 0.000000000000000000, 0.000000000000000000, 1.000000000000000000 ) ) ;
#14186=VECTOR ( 'NONE', #13019, 1000.000000000000000 ) ;
#14199=ORIENTED_EDGE ( 'NONE', *, *, #8161, .F. ) ;
#14200=LINE ( 'NONE', #12105, #10558 ) ;
#14207=EDGE_CURVE ( 'NONE', #9120, #3114, #1086, .T. ) ;
#14209=DIRECTION ( 'NONE',  ( -0.000000000000000000, -1.000000000000000000, -0.000000000000000000 ) ) ;
#14213=LINE ( 'NONE', #3279, #8666 ) ;
#14217=EDGE_CURVE ( 'NONE', #2121, #3167, #10013, .T. ) ;
#14219=VERTEX_POINT ( 'NONE', #13270 ) ;
#14228=DIRECTION ( 'NONE',  ( -0.000000000000000000, -0.000000000000000000, 1.000000000000000000 ) ) ;
#14236=ORIENTED_EDGE ( 'NONE', *, *, #13846, .T. ) ;
#14238=DIRECTION ( 'NONE',  ( -0.000000000000000000, 1.000000000000000000, -0.000000000000000000 ) ) ;
#14243=CIRCLE ( 'NONE', #1027, 2.649999999999985700 ) ;
#14244=EDGE_LOOP ( 'NONE', ( #6301, #4711, #5267 ) ) ;
#14246=CARTESIAN_POINT ( 'NONE',  ( 238.9999999999999432, -85.00000000000007105, 180.0000000000000000 ) ) ;
#14249=ORIENTED_EDGE ( 'NONE', *, *, #6715, .T. ) ;
#14253=VERTEX_POINT ( 'NONE', #12115 ) ;
#14256=VERTEX_POINT ( 'NONE', #2028 ) ;
#14265=CIRCLE ( 'NONE', #13346, 2.649999999999985700 ) ;
#14266=EDGE_LOOP ( 'NONE', ( #9328, #5265, #1117, #13569 ) ) ;
#14287=VECTOR ( 'NONE', #9823, 1000.000000000000000 ) ;
#14292=FACE_OUTER_BOUND ( 'NONE', #5944, .T. ) ;
#14297=AXIS2_PLACEMENT_3D ( 'NONE', #11833, #6318, #3064 ) ;
#14299=DIRECTION ( 'NONE',  ( 0.000000000000000000, 0.000000000000000000, -1.000000000000000000 ) ) ;
#14303=VECTOR ( 'NONE', #11972, 1000.000000000000000 ) ;
#14306=ORIENTED_EDGE ( 'NONE', *, *, #10530, .T. ) ;
#14383=COLOUR_RGB('Dark Blue',0.08,0.2,0.34);
#14384=FILL_AREA_STYLE_COLOUR('',#14383);
#14385=FILL_AREA_STYLE('',(#14384));
#14386=SURFACE_STYLE_FILL_AREA(#14385);
#14387=SURFACE_SIDE_STYLE('',(#14386));
#14388=SURFACE_STYLE_USAGE(.BOTH.,#14387);
#14389=PRESENTATION_STYLE_ASSIGNMENT((#14388));
ENDSEC;
END-ISO-10303-21;
